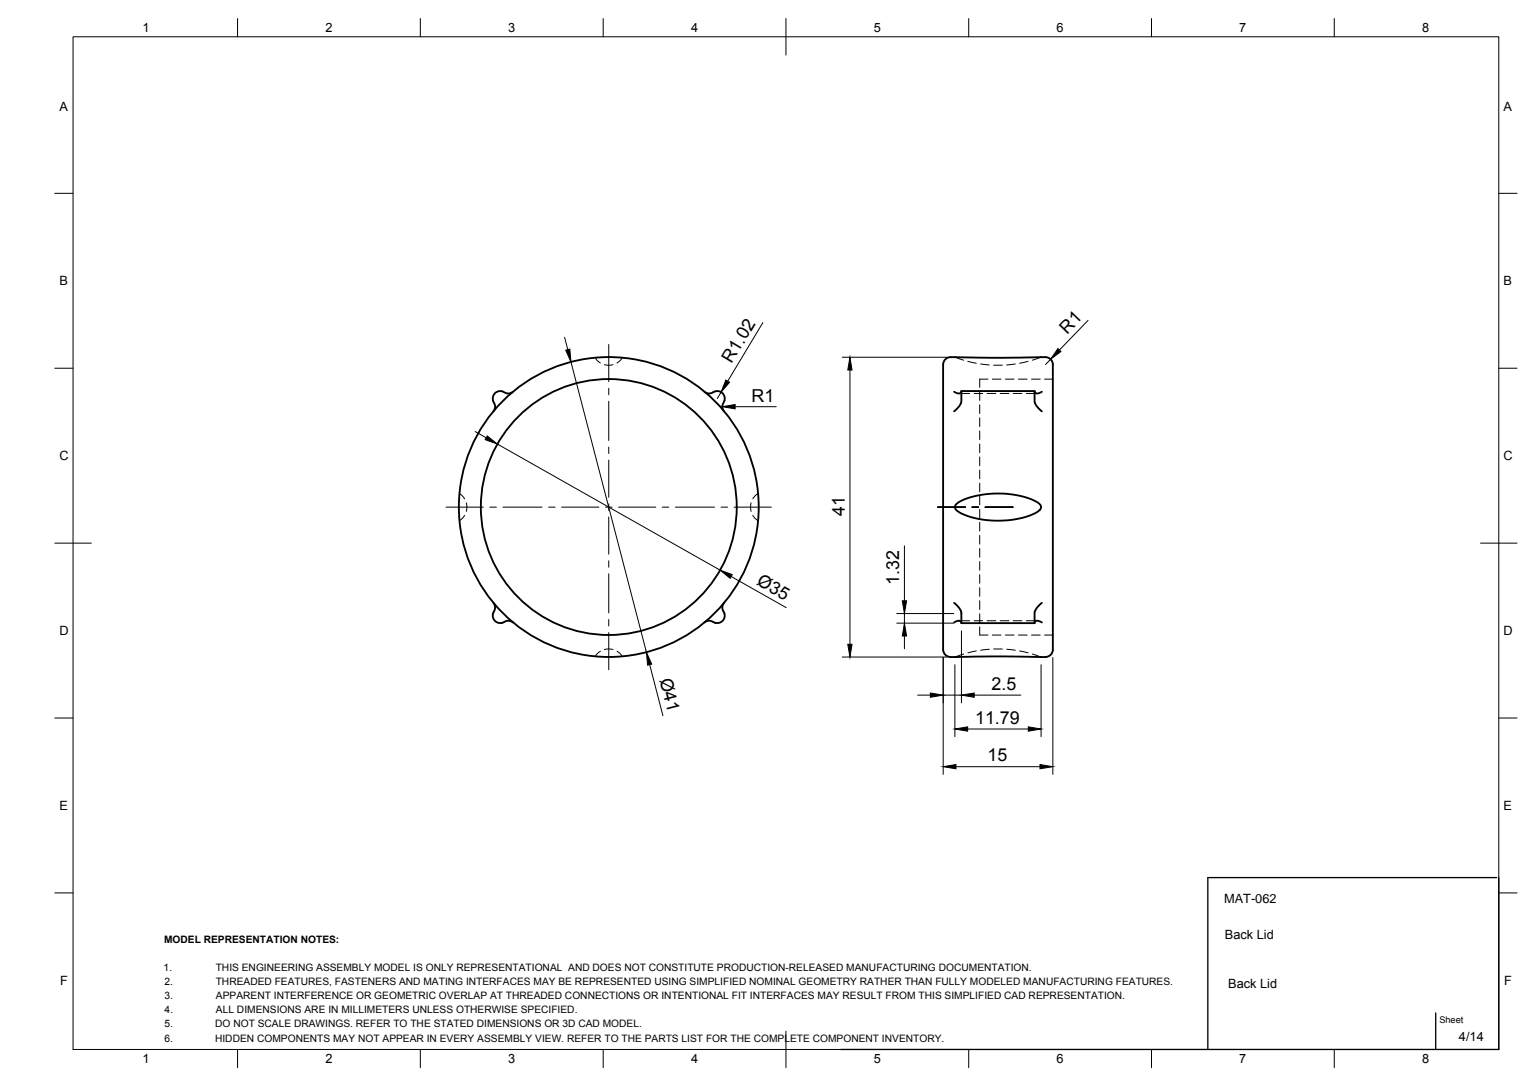
ISO-10303-21;
HEADER;
/* Generated by software containing ST-Developer
 * from STEP Tools, Inc. (www.steptools.com) 
 */

FILE_DESCRIPTION(
/* description */ (''),
/* implementation_level */ '2;1');

FILE_NAME(
/* name */ 'Back Lid.step',
/* time_stamp */ '2026-10-24T10:18:25-07:00',
/* author */ (''),
/* organization */ (''),
/* preprocessor_version */ 'ST-DEVELOPER v20.2',
/* originating_system */ 'Autodesk Translation Framework v15.15.0.0',
/* authorisation */ '');

FILE_SCHEMA (('AUTOMOTIVE_DESIGN { 1 0 10303 214 3 1 1 }'));
ENDSEC;

DATA;
#10=MECHANICAL_DESIGN_GEOMETRIC_PRESENTATION_REPRESENTATION('',(#248),#14125);
#199=TOROIDAL_SURFACE('',#6365,21.5,1.);
#200=TOROIDAL_SURFACE('',#6366,21.5,1.);
#201=TOROIDAL_SURFACE('',#6390,21.5,1.);
#202=TOROIDAL_SURFACE('',#6391,21.5,1.);
#203=TOROIDAL_SURFACE('',#6394,21.5,1.);
#204=TOROIDAL_SURFACE('',#6395,21.5,1.);
#205=TOROIDAL_SURFACE('',#6398,21.5,1.);
#206=TOROIDAL_SURFACE('',#6399,21.5,1.);
#207=TOROIDAL_SURFACE('',#6401,19.5,1.);
#208=TOROIDAL_SURFACE('',#6403,19.5,1.);
#219=(
BOUNDED_SURFACE()
B_SPLINE_SURFACE(2,2,((#10435,#10436,#10437,#10438,#10439),(#10440,#10441,
#10442,#10443,#10444),(#10445,#10446,#10447,#10448,#10449)),
 .UNSPECIFIED.,.F.,.F.,.F.)
B_SPLINE_SURFACE_WITH_KNOTS((3,3),(3,2,3),(-0.372145961557786,0.372122372471418),
(-2.5862005619648,-1.57539112175776,-0.564581681550713),.UNSPECIFIED.)
GEOMETRIC_REPRESENTATION_ITEM()
RATIONAL_B_SPLINE_SURFACE(((1.,0.874978596158143,1.,0.874978596158143,1.),
(0.931553475244656,0.815089352015808,0.931553475244656,0.815089352015808,
0.931553475244656),(1.,0.874978596158143,1.,0.874978596158143,1.)))
REPRESENTATION_ITEM('')
SURFACE()
);
#220=(
BOUNDED_SURFACE()
B_SPLINE_SURFACE(2,2,((#10450,#10451,#10452,#10453,#10454),(#10455,#10456,
#10457,#10458,#10459),(#10460,#10461,#10462,#10463,#10464)),
 .UNSPECIFIED.,.F.,.F.,.F.)
B_SPLINE_SURFACE_WITH_KNOTS((3,3),(3,2,3),(-0.372145961557785,0.372122372471416),
(-1.01540423516984,-0.00459479496282911,1.00621464524418),.UNSPECIFIED.)
GEOMETRIC_REPRESENTATION_ITEM()
RATIONAL_B_SPLINE_SURFACE(((1.,0.874978596158151,1.,0.874978596158151,1.),
(0.931553475244656,0.815089352015816,0.931553475244656,0.815089352015816,
0.931553475244656),(1.,0.874978596158151,1.,0.874978596158151,1.)))
REPRESENTATION_ITEM('')
SURFACE()
);
#221=(
BOUNDED_SURFACE()
B_SPLINE_SURFACE(2,2,((#10465,#10466,#10467,#10468,#10469),(#10470,#10471,
#10472,#10473,#10474),(#10475,#10476,#10477,#10478,#10479)),
 .UNSPECIFIED.,.F.,.F.,.F.)
B_SPLINE_SURFACE_WITH_KNOTS((3,3),(3,2,3),(-0.372145961557786,0.372122372471418),
(0.555392091624955,1.56620153183202,2.57701097203908),.UNSPECIFIED.)
GEOMETRIC_REPRESENTATION_ITEM()
RATIONAL_B_SPLINE_SURFACE(((1.,0.874978596158138,1.,0.874978596158138,1.),
(0.931553475244654,0.815089352015803,0.931553475244654,0.815089352015803,
0.931553475244654),(1.,0.874978596158138,1.,0.874978596158138,1.)))
REPRESENTATION_ITEM('')
SURFACE()
);
#222=(
BOUNDED_SURFACE()
B_SPLINE_SURFACE(2,2,((#10480,#10481,#10482,#10483,#10484),(#10485,#10486,
#10487,#10488,#10489),(#10490,#10491,#10492,#10493,#10494)),
 .UNSPECIFIED.,.F.,.F.,.F.)
B_SPLINE_SURFACE_WITH_KNOTS((3,3),(3,2,3),(-0.371934671474245,0.371934671474244),
(-1.01080944020701,0.,1.01080944020701),.UNSPECIFIED.)
GEOMETRIC_REPRESENTATION_ITEM()
RATIONAL_B_SPLINE_SURFACE(((1.,0.87497859615815,1.,0.87497859615815,1.),
(0.93162599415309,0.815152804508512,0.93162599415309,0.815152804508512,
0.93162599415309),(1.,0.87497859615815,1.,0.87497859615815,1.)))
REPRESENTATION_ITEM('')
SURFACE()
);
#228=SHAPE_REPRESENTATION_RELATIONSHIP('SRR','None',#14201,#238);
#238=ADVANCED_BREP_SHAPE_REPRESENTATION('',(#267),#14115);
#248=STYLED_ITEM('',(#14263),#267);
#267=MANIFOLD_SOLID_BREP('Back Lid',#6135);
#319=B_SPLINE_CURVE_WITH_KNOTS('',3,(#10199,#10200,#10201,#10202,#10203,
#10204,#10205,#10206),.UNSPECIFIED.,.F.,.F.,(4,2,2,4),(-1.01270550863141,
-0.972225883052009,-0.93592471729076,-0.9302261633243),.UNSPECIFIED.);
#320=B_SPLINE_CURVE_WITH_KNOTS('',3,(#10208,#10209,#10210,#10211,#10212,
#10213,#10214,#10215,#10216,#10217,#10218,#10219,#10220,#10221,#10222,#10223,
#10224,#10225,#10226,#10227,#10228,#10229),.UNSPECIFIED.,.F.,.F.,(4,2,2,
2,2,2,2,2,2,2,4),(0.770301299294677,0.776837516381544,0.810179859704117,
0.863854547164407,0.965601485426607,1.16658222290299,1.71041595764289,2.04547866914785,
2.21675572625692,2.31744906128486,2.32707423972487),.UNSPECIFIED.);
#321=B_SPLINE_CURVE_WITH_KNOTS('',3,(#10235,#10236,#10237,#10238,#10239,
#10240,#10241,#10242,#10243,#10244,#10245,#10246,#10247,#10248,#10249,#10250,
#10251,#10252,#10253,#10254,#10255,#10256,#10257,#10258,#10259),
 .UNSPECIFIED.,.F.,.F.,(4,2,2,2,2,3,2,2,2,2,2,4),(-0.9302261633243,-0.897559179923855,
-0.841033612998941,-0.72014052841894,-0.534875041413907,0.,0.287237711284631,
0.543909079429507,0.657892073847931,0.715678915934471,0.748705009105826,
0.770301299294677),.UNSPECIFIED.);
#322=B_SPLINE_CURVE_WITH_KNOTS('',3,(#10293,#10294,#10295,#10296,#10297,
#10298,#10299,#10300,#10301,#10302,#10303,#10304,#10305,#10306,#10307,#10308,
#10309,#10310,#10311,#10312,#10313,#10314,#10315,#10316,#10317,#10318,#10319,
#10320,#10321,#10322,#10323,#10324,#10325,#10326,#10327,#10328,#10329,#10330,
#10331,#10332,#10333,#10334,#10335,#10336),.UNSPECIFIED.,.T.,.F.,(4,2,2,
2,2,2,2,2,2,2,2,2,2,2,2,2,2,2,2,2,2,4),(-3.33977974833692,-3.05254203705232,
-2.79587066890727,-2.68188767448872,-2.62410083240212,-2.59107473923068,
-2.56294223195498,-2.52959988863245,-2.47592520117237,-2.37417826291126,
-2.17319752543706,-1.62936379070288,-1.29430107920164,-1.12302402209434,
-1.02233068706724,-0.972225883048282,-0.935924717287512,-0.897559179921191,
-0.841033612997187,-0.720140528418584,-0.534875041413949,0.),
 .UNSPECIFIED.);
#323=B_SPLINE_CURVE_WITH_KNOTS('',3,(#10338,#10339,#10340,#10341,#10342,
#10343,#10344,#10345,#10346,#10347,#10348,#10349,#10350,#10351,#10352,#10353,
#10354,#10355,#10356,#10357,#10358,#10359,#10360,#10361,#10362,#10363,#10364,
#10365,#10366,#10367,#10368,#10369,#10370,#10371,#10372,#10373,#10374,#10375,
#10376,#10377,#10378,#10379,#10380,#10381),.UNSPECIFIED.,.T.,.F.,(4,2,2,
2,2,2,2,2,2,2,2,2,2,2,2,2,2,2,2,2,2,4),(-3.3397797483622,-3.05254203707762,
-2.79587066893242,-2.68188767451365,-2.62410083242683,-2.5910747392553,
-2.5629422319795,-2.52959988865681,-2.47592520119621,-2.37417826293345,
-2.17319752545607,-1.62936379071395,-1.29430107920719,-1.1230240220981,
-1.02233068707054,-0.972225883051298,-0.93592471729009,-0.89755917992317,
-0.841033612998203,-0.720140528418294,-0.534875041413579,0.),
 .UNSPECIFIED.);
#324=B_SPLINE_CURVE_WITH_KNOTS('',3,(#10383,#10384,#10385,#10386,#10387,
#10388,#10389,#10390,#10391,#10392,#10393,#10394,#10395,#10396,#10397,#10398,
#10399,#10400,#10401,#10402,#10403,#10404,#10405,#10406,#10407,#10408,#10409,
#10410,#10411,#10412,#10413,#10414,#10415,#10416,#10417,#10418,#10419,#10420,
#10421,#10422,#10423,#10424,#10425,#10426),.UNSPECIFIED.,.T.,.F.,(4,2,2,
2,2,2,2,2,2,2,2,2,2,2,2,2,2,2,2,2,2,4),(-3.3397797483903,-3.05254203710569,
-2.79587066896086,-2.68188767454252,-2.62410083245608,-2.59107473928483,
-2.56294223200934,-2.52959988868709,-2.47592520122646,-2.37417826296174,
-2.17319752548078,-1.62936379072977,-1.29430107921846,-1.12302402210607,
-1.02233068707609,-0.972225883055856,-0.935924717293985,-0.897559179926439,
-0.841033613000712,-0.720140528419696,-0.534875041414283,0.),
 .UNSPECIFIED.);
#325=B_SPLINE_CURVE_WITH_KNOTS('',3,(#10500,#10501,#10502,#10503,#10504,
#10505),.UNSPECIFIED.,.F.,.F.,(4,2,4),(0.661047189651573,0.682893822496354,
0.69260663288377),.UNSPECIFIED.);
#326=B_SPLINE_CURVE_WITH_KNOTS('',3,(#10509,#10510,#10511,#10512,#10513,
#10514),.UNSPECIFIED.,.F.,.F.,(4,2,4),(0.954385955540414,0.955688960187291,
0.983990255335198),.UNSPECIFIED.);
#327=B_SPLINE_CURVE_WITH_KNOTS('',3,(#10518,#10519,#10520,#10521,#10522,
#10523),.UNSPECIFIED.,.F.,.F.,(4,2,4),(0.11431583352954,0.135832218753253,
0.145774815807224),.UNSPECIFIED.);
#328=B_SPLINE_CURVE_WITH_KNOTS('',3,(#10526,#10527,#10528,#10529,#10530,
#10531),.UNSPECIFIED.,.F.,.F.,(4,2,4),(0.406957049146252,0.408029153839697,
0.43652027355868),.UNSPECIFIED.);
#329=B_SPLINE_CURVE_WITH_KNOTS('',3,(#10537,#10538,#10539,#10540,#10541,
#10542,#10543,#10544,#10545,#10546),.UNSPECIFIED.,.F.,.F.,(4,2,2,2,4),(-0.178698063821344,
-0.13526955955559,-0.076624980274606,0.,0.000624348927189005),
 .UNSPECIFIED.);
#330=B_SPLINE_CURVE_WITH_KNOTS('',3,(#10547,#10548,#10549,#10550,#10551,
#10552,#10553,#10554,#10555,#10556),.UNSPECIFIED.,.F.,.F.,(4,2,2,2,4),(0.221433756193381,
0.257003031040665,0.305034737267452,0.367792942517405,0.3683043034075),
 .UNSPECIFIED.);
#331=B_SPLINE_CURVE_WITH_KNOTS('',3,(#10558,#10559,#10560,#10561,#10562,
#10563,#10564,#10565,#10566,#10567),.UNSPECIFIED.,.F.,.F.,(4,2,2,2,4),(-0.178698063657826,
-0.135269559443281,-0.0766249802302674,0.,0.000624348926984052),
 .UNSPECIFIED.);
#332=B_SPLINE_CURVE_WITH_KNOTS('',3,(#10569,#10570,#10571,#10572,#10573,
#10574,#10575,#10576,#10577,#10578),.UNSPECIFIED.,.F.,.F.,(4,2,2,2,4),(0.22143375619356,
0.257003031040236,0.305034737266783,0.367792942534155,0.36830430342492),
 .UNSPECIFIED.);
#333=B_SPLINE_CURVE_WITH_KNOTS('',3,(#10585,#10586,#10587,#10588,#10589,
#10590),.UNSPECIFIED.,.F.,.F.,(4,2,4),(0.661047189631137,0.682893822475484,
0.692606632862655),.UNSPECIFIED.);
#334=B_SPLINE_CURVE_WITH_KNOTS('',3,(#10594,#10595,#10596,#10597,#10598,
#10599),.UNSPECIFIED.,.F.,.F.,(4,2,4),(0.954385955875588,0.955688960523108,
0.983990255684603),.UNSPECIFIED.);
#335=B_SPLINE_CURVE_WITH_KNOTS('',3,(#10603,#10604,#10605,#10606,#10607,
#10608),.UNSPECIFIED.,.F.,.F.,(4,2,4),(0.11431583355748,0.135832218786672,
0.145774815843186),.UNSPECIFIED.);
#336=B_SPLINE_CURVE_WITH_KNOTS('',3,(#10611,#10612,#10613,#10614,#10615,
#10616),.UNSPECIFIED.,.F.,.F.,(4,2,4),(0.406957049130622,0.408029153824045,
0.436520273542523),.UNSPECIFIED.);
#337=B_SPLINE_CURVE_WITH_KNOTS('',3,(#10626,#10627,#10628,#10629,#10630,
#10631),.UNSPECIFIED.,.F.,.F.,(4,2,4),(0.661047189621191,0.682893822464398,
0.692606632851314),.UNSPECIFIED.);
#338=B_SPLINE_CURVE_WITH_KNOTS('',3,(#10635,#10636,#10637,#10638,#10639,
#10640),.UNSPECIFIED.,.F.,.F.,(4,2,4),(0.954385955650832,0.95568896029806,
0.983990255452134),.UNSPECIFIED.);
#339=B_SPLINE_CURVE_WITH_KNOTS('',3,(#10644,#10645,#10646,#10647,#10648,
#10649),.UNSPECIFIED.,.F.,.F.,(4,2,4),(0.114315833531678,0.135832218756235,
0.145774815810657),.UNSPECIFIED.);
#340=B_SPLINE_CURVE_WITH_KNOTS('',3,(#10652,#10653,#10654,#10655,#10656,
#10657),.UNSPECIFIED.,.F.,.F.,(4,2,4),(0.406957049123385,0.408029153816832,
0.43652027353595),.UNSPECIFIED.);
#341=B_SPLINE_CURVE_WITH_KNOTS('',3,(#10667,#10668,#10669,#10670,#10671,
#10672),.UNSPECIFIED.,.F.,.F.,(4,2,4),(0.661047189700789,0.682893822549002,
0.692606632937976),.UNSPECIFIED.);
#342=B_SPLINE_CURVE_WITH_KNOTS('',3,(#10676,#10677,#10678,#10679,#10680,
#10681),.UNSPECIFIED.,.F.,.F.,(4,2,4),(0.954385955972242,0.955688960619816,
0.983990255786846),.UNSPECIFIED.);
#343=B_SPLINE_CURVE_WITH_KNOTS('',3,(#10685,#10686,#10687,#10688,#10689,
#10690),.UNSPECIFIED.,.F.,.F.,(4,2,4),(0.114315833560946,0.135832218791008,
0.145774815847966),.UNSPECIFIED.);
#344=B_SPLINE_CURVE_WITH_KNOTS('',3,(#10693,#10694,#10695,#10696,#10697,
#10698),.UNSPECIFIED.,.F.,.F.,(4,2,4),(0.406957049170082,0.408029153863569,
0.436520273584039),.UNSPECIFIED.);
#345=B_SPLINE_CURVE_WITH_KNOTS('',3,(#10704,#10705,#10706,#10707,#10708,
#10709,#10710,#10711,#10712,#10713),.UNSPECIFIED.,.F.,.F.,(4,2,2,2,4),(-0.17869806353704,
-0.135269559359834,-0.0766249801970823,0.,0.000624348926732177),
 .UNSPECIFIED.);
#346=B_SPLINE_CURVE_WITH_KNOTS('',3,(#10714,#10715,#10716,#10717,#10718,
#10719,#10720,#10721,#10722,#10723),.UNSPECIFIED.,.F.,.F.,(4,2,2,2,4),(0.221433756192697,
0.257003031038445,0.305034737264325,0.3677929425703,0.368304303461073),
 .UNSPECIFIED.);
#347=B_SPLINE_CURVE_WITH_KNOTS('',3,(#10725,#10726,#10727,#10728,#10729,
#10730,#10731,#10732,#10733,#10734),.UNSPECIFIED.,.F.,.F.,(4,2,2,2,4),(-0.178698063770044,
-0.135269559520182,-0.0766249802604931,0.,0.000624348926843672),
 .UNSPECIFIED.);
#348=B_SPLINE_CURVE_WITH_KNOTS('',3,(#10736,#10737,#10738,#10739,#10740,
#10741,#10742,#10743,#10744,#10745),.UNSPECIFIED.,.F.,.F.,(4,2,2,2,4),(0.221433756193478,
0.257003031040149,0.305034737266569,0.367792942538401,0.368304303428461),
 .UNSPECIFIED.);
#349=B_SPLINE_CURVE_WITH_KNOTS('',3,(#10748,#10749,#10750,#10751,#10752,
#10753,#10754,#10755,#10756,#10757),.UNSPECIFIED.,.F.,.F.,(4,2,2,2,4),(-0.178698063553284,
-0.135269559371072,-0.0766249802015666,0.,0.000624348926677296),
 .UNSPECIFIED.);
#350=B_SPLINE_CURVE_WITH_KNOTS('',3,(#10758,#10759,#10760,#10761,#10762,
#10763,#10764,#10765,#10766,#10767),.UNSPECIFIED.,.F.,.F.,(4,2,2,2,4),(0.221433756192838,
0.25700303103897,0.305034737265084,0.367792942555533,0.368304303445851),
 .UNSPECIFIED.);
#351=B_SPLINE_CURVE_WITH_KNOTS('',3,(#10769,#10770,#10771,#10772,#10773,
#10774,#10775,#10776,#10777,#10778),.UNSPECIFIED.,.F.,.F.,(4,2,2,2,4),(-0.178698063553173,
-0.135269559370956,-0.0766249802014978,0.,0.000624348926817562),
 .UNSPECIFIED.);
#352=B_SPLINE_CURVE_WITH_KNOTS('',3,(#10780,#10781,#10782,#10783,#10784,
#10785,#10786,#10787,#10788,#10789),.UNSPECIFIED.,.F.,.F.,(4,2,2,2,4),(0.221433756193333,
0.25700303103906,0.305034737264906,0.367792942572609,0.368304303463133),
 .UNSPECIFIED.);
#353=B_SPLINE_CURVE_WITH_KNOTS('',3,(#10792,#10793,#10794,#10795,#10796,
#10797,#10798,#10799,#10800,#10801),.UNSPECIFIED.,.F.,.F.,(4,2,2,2,4),(-0.178698063530463,
-0.135269559355353,-0.0766249801953056,0.,0.000624348926771406),
 .UNSPECIFIED.);
#354=B_SPLINE_CURVE_WITH_KNOTS('',3,(#10802,#10803,#10804,#10805,#10806,
#10807,#10808,#10809,#10810,#10811),.UNSPECIFIED.,.F.,.F.,(4,2,2,2,4),(0.221433756193692,
0.2570030310401,0.30503473726647,0.367792942548679,0.368304303439319),
 .UNSPECIFIED.);
#355=B_SPLINE_CURVE_WITH_KNOTS('',3,(#10813,#10814,#10815,#10816,#10817,
#10818,#10819,#10820,#10821,#10822),.UNSPECIFIED.,.F.,.F.,(4,2,2,2,4),(-0.178698063395802,
-0.135269559262804,-0.0766249801587596,0.,0.00062434892634055),
 .UNSPECIFIED.);
#356=B_SPLINE_CURVE_WITH_KNOTS('',3,(#10824,#10825,#10826,#10827,#10828,
#10829,#10830,#10831,#10832,#10833),.UNSPECIFIED.,.F.,.F.,(4,2,2,2,4),(0.221433756192834,
0.257003031038388,0.305034737264263,0.367792942576978,0.368304303467952),
 .UNSPECIFIED.);
#499=CYLINDRICAL_SURFACE('',#6339,20.5);
#500=CYLINDRICAL_SURFACE('',#6357,1.02425693042952);
#501=CYLINDRICAL_SURFACE('',#6364,1.);
#502=CYLINDRICAL_SURFACE('',#6367,1.);
#503=CYLINDRICAL_SURFACE('',#6368,1.02425693042952);
#504=CYLINDRICAL_SURFACE('',#6375,1.02425693042952);
#505=CYLINDRICAL_SURFACE('',#6382,1.02425693042952);
#506=CYLINDRICAL_SURFACE('',#6389,1.);
#507=CYLINDRICAL_SURFACE('',#6392,1.);
#508=CYLINDRICAL_SURFACE('',#6393,1.);
#509=CYLINDRICAL_SURFACE('',#6396,1.);
#510=CYLINDRICAL_SURFACE('',#6397,1.);
#511=CYLINDRICAL_SURFACE('',#6400,1.);
#512=CYLINDRICAL_SURFACE('',#6405,17.5);
#646=FACE_BOUND('',#1156,.T.);
#647=FACE_BOUND('',#1157,.T.);
#648=FACE_BOUND('',#1158,.T.);
#649=FACE_BOUND('',#1159,.T.);
#650=FACE_BOUND('',#1160,.T.);
#651=FACE_BOUND('',#1161,.T.);
#652=FACE_BOUND('',#1162,.T.);
#653=FACE_BOUND('',#1165,.T.);
#783=FACE_OUTER_BOUND('',#1155,.T.);
#784=FACE_OUTER_BOUND('',#1163,.T.);
#785=FACE_OUTER_BOUND('',#1164,.T.);
#786=FACE_OUTER_BOUND('',#1166,.T.);
#787=FACE_OUTER_BOUND('',#1167,.T.);
#788=FACE_OUTER_BOUND('',#1168,.T.);
#789=FACE_OUTER_BOUND('',#1169,.T.);
#790=FACE_OUTER_BOUND('',#1170,.T.);
#791=FACE_OUTER_BOUND('',#1171,.T.);
#792=FACE_OUTER_BOUND('',#1172,.T.);
#793=FACE_OUTER_BOUND('',#1173,.T.);
#794=FACE_OUTER_BOUND('',#1174,.T.);
#795=FACE_OUTER_BOUND('',#1175,.T.);
#796=FACE_OUTER_BOUND('',#1176,.T.);
#797=FACE_OUTER_BOUND('',#1177,.T.);
#798=FACE_OUTER_BOUND('',#1178,.T.);
#799=FACE_OUTER_BOUND('',#1179,.T.);
#800=FACE_OUTER_BOUND('',#1180,.T.);
#801=FACE_OUTER_BOUND('',#1181,.T.);
#802=FACE_OUTER_BOUND('',#1182,.T.);
#803=FACE_OUTER_BOUND('',#1183,.T.);
#804=FACE_OUTER_BOUND('',#1184,.T.);
#805=FACE_OUTER_BOUND('',#1185,.T.);
#806=FACE_OUTER_BOUND('',#1186,.T.);
#807=FACE_OUTER_BOUND('',#1187,.T.);
#808=FACE_OUTER_BOUND('',#1188,.T.);
#809=FACE_OUTER_BOUND('',#1189,.T.);
#810=FACE_OUTER_BOUND('',#1190,.T.);
#811=FACE_OUTER_BOUND('',#1191,.T.);
#812=FACE_OUTER_BOUND('',#1192,.T.);
#813=FACE_OUTER_BOUND('',#1193,.T.);
#814=FACE_OUTER_BOUND('',#1194,.T.);
#815=FACE_OUTER_BOUND('',#1195,.T.);
#816=FACE_OUTER_BOUND('',#1196,.T.);
#817=FACE_OUTER_BOUND('',#1197,.T.);
#818=FACE_OUTER_BOUND('',#1198,.T.);
#819=FACE_OUTER_BOUND('',#1199,.T.);
#820=FACE_OUTER_BOUND('',#1200,.T.);
#821=FACE_OUTER_BOUND('',#1201,.T.);
#1155=EDGE_LOOP('',(#4221,#4222,#4223,#4224,#4225,#4226,#4227,#4228,#4229,
#4230,#4231));
#1156=EDGE_LOOP('',(#4232,#4233,#4234,#4235));
#1157=EDGE_LOOP('',(#4236,#4237,#4238,#4239));
#1158=EDGE_LOOP('',(#4240,#4241,#4242,#4243));
#1159=EDGE_LOOP('',(#4244,#4245,#4246,#4247));
#1160=EDGE_LOOP('',(#4248));
#1161=EDGE_LOOP('',(#4249));
#1162=EDGE_LOOP('',(#4250));
#1163=EDGE_LOOP('',(#4251));
#1164=EDGE_LOOP('',(#4252));
#1165=EDGE_LOOP('',(#4253));
#1166=EDGE_LOOP('',(#4254));
#1167=EDGE_LOOP('',(#4255));
#1168=EDGE_LOOP('',(#4256));
#1169=EDGE_LOOP('',(#4257,#4258,#4259));
#1170=EDGE_LOOP('',(#4260,#4261,#4262,#4263,#4264,#4265,#4266,#4267));
#1171=EDGE_LOOP('',(#4268,#4269));
#1172=EDGE_LOOP('',(#4270,#4271));
#1173=EDGE_LOOP('',(#4272,#4273,#4274,#4275));
#1174=EDGE_LOOP('',(#4276,#4277,#4278,#4279,#4280,#4281));
#1175=EDGE_LOOP('',(#4282,#4283,#4284,#4285,#4286,#4287));
#1176=EDGE_LOOP('',(#4288,#4289,#4290,#4291));
#1177=EDGE_LOOP('',(#4292,#4293,#4294,#4295,#4296,#4297,#4298,#4299));
#1178=EDGE_LOOP('',(#4300,#4301));
#1179=EDGE_LOOP('',(#4302,#4303));
#1180=EDGE_LOOP('',(#4304,#4305,#4306,#4307,#4308,#4309,#4310,#4311));
#1181=EDGE_LOOP('',(#4312,#4313));
#1182=EDGE_LOOP('',(#4314,#4315));
#1183=EDGE_LOOP('',(#4316,#4317,#4318,#4319,#4320,#4321,#4322,#4323));
#1184=EDGE_LOOP('',(#4324,#4325));
#1185=EDGE_LOOP('',(#4326,#4327));
#1186=EDGE_LOOP('',(#4328,#4329,#4330,#4331));
#1187=EDGE_LOOP('',(#4332,#4333,#4334,#4335,#4336,#4337));
#1188=EDGE_LOOP('',(#4338,#4339,#4340,#4341,#4342,#4343));
#1189=EDGE_LOOP('',(#4344,#4345,#4346,#4347));
#1190=EDGE_LOOP('',(#4348,#4349,#4350,#4351));
#1191=EDGE_LOOP('',(#4352,#4353,#4354,#4355,#4356,#4357));
#1192=EDGE_LOOP('',(#4358,#4359,#4360,#4361,#4362,#4363));
#1193=EDGE_LOOP('',(#4364,#4365,#4366,#4367));
#1194=EDGE_LOOP('',(#4368,#4369,#4370,#4371));
#1195=EDGE_LOOP('',(#4372,#4373,#4374,#4375,#4376,#4377));
#1196=EDGE_LOOP('',(#4378,#4379,#4380,#4381,#4382,#4383));
#1197=EDGE_LOOP('',(#4384,#4385,#4386,#4387));
#1198=EDGE_LOOP('',(#4388,#4389,#4390,#4391,#4392));
#1199=EDGE_LOOP('',(#4393,#4394,#4395,#4396,#4397));
#1200=EDGE_LOOP('',(#4398,#4399,#4400,#4401));
#1201=EDGE_LOOP('',(#4402));
#1580=CIRCLE('',#6340,20.5);
#1581=CIRCLE('',#6341,20.5);
#1582=CIRCLE('',#6342,20.5);
#1583=CIRCLE('',#6343,20.5);
#1584=CIRCLE('',#6344,20.5);
#1585=CIRCLE('',#6345,20.5);
#1586=CIRCLE('',#6346,20.5);
#1587=CIRCLE('',#6347,20.5);
#1588=CIRCLE('',#6348,20.5);
#1589=CIRCLE('',#6349,20.5);
#1590=CIRCLE('',#6350,20.5);
#1591=CIRCLE('',#6351,20.5);
#1592=CIRCLE('',#6353,19.5);
#1593=CIRCLE('',#6355,19.5);
#1594=CIRCLE('',#6356,17.5);
#1595=CIRCLE('',#6358,1.02425693042952);
#1596=CIRCLE('',#6359,1.02425693042952);
#1597=CIRCLE('',#6361,21.5);
#1598=CIRCLE('',#6363,21.5);
#1599=CIRCLE('',#6369,1.02425693042952);
#1600=CIRCLE('',#6370,1.02425693042952);
#1601=CIRCLE('',#6372,21.5);
#1602=CIRCLE('',#6374,21.5);
#1603=CIRCLE('',#6376,1.02425693042952);
#1604=CIRCLE('',#6377,1.02425693042952);
#1605=CIRCLE('',#6379,21.5);
#1606=CIRCLE('',#6381,21.5);
#1607=CIRCLE('',#6383,1.02425693042952);
#1608=CIRCLE('',#6384,1.02425693042952);
#1609=CIRCLE('',#6386,21.5);
#1610=CIRCLE('',#6388,21.5);
#1611=CIRCLE('',#6402,1.);
#1612=CIRCLE('',#6404,1.);
#1613=CIRCLE('',#6406,17.5);
#1869=LINE('',#10197,#2257);
#1870=LINE('',#10231,#2258);
#1871=LINE('',#10262,#2259);
#1872=LINE('',#10266,#2260);
#1873=LINE('',#10270,#2261);
#1874=LINE('',#10274,#2262);
#1875=LINE('',#10278,#2263);
#1876=LINE('',#10282,#2264);
#1877=LINE('',#10286,#2265);
#1878=LINE('',#10290,#2266);
#1879=LINE('',#10507,#2267);
#1880=LINE('',#10525,#2268);
#1881=LINE('',#10592,#2269);
#1882=LINE('',#10610,#2270);
#1883=LINE('',#10633,#2271);
#1884=LINE('',#10651,#2272);
#1885=LINE('',#10674,#2273);
#1886=LINE('',#10692,#2274);
#1887=LINE('',#10841,#2275);
#2257=VECTOR('',#7141,20.5);
#2258=VECTOR('',#7142,20.5);
#2259=VECTOR('',#7147,12.);
#2260=VECTOR('',#7150,12.);
#2261=VECTOR('',#7153,12.);
#2262=VECTOR('',#7156,12.);
#2263=VECTOR('',#7159,12.);
#2264=VECTOR('',#7162,12.);
#2265=VECTOR('',#7165,12.);
#2266=VECTOR('',#7168,12.);
#2267=VECTOR('',#7185,10.0757988598381);
#2268=VECTOR('',#7188,10.0757988598381);
#2269=VECTOR('',#7209,10.0757988598381);
#2270=VECTOR('',#7212,10.0757988598381);
#2271=VECTOR('',#7225,10.0757988598381);
#2272=VECTOR('',#7228,10.0757988598381);
#2273=VECTOR('',#7241,10.0757988598381);
#2274=VECTOR('',#7244,10.0757988598381);
#2275=VECTOR('',#7287,17.5);
#2659=VERTEX_POINT('',#10192);
#2660=VERTEX_POINT('',#10193);
#2661=VERTEX_POINT('',#10196);
#2662=VERTEX_POINT('',#10198);
#2663=VERTEX_POINT('',#10207);
#2664=VERTEX_POINT('',#10230);
#2665=VERTEX_POINT('',#10232);
#2666=VERTEX_POINT('',#10260);
#2667=VERTEX_POINT('',#10261);
#2668=VERTEX_POINT('',#10263);
#2669=VERTEX_POINT('',#10265);
#2670=VERTEX_POINT('',#10268);
#2671=VERTEX_POINT('',#10269);
#2672=VERTEX_POINT('',#10271);
#2673=VERTEX_POINT('',#10273);
#2674=VERTEX_POINT('',#10276);
#2675=VERTEX_POINT('',#10277);
#2676=VERTEX_POINT('',#10279);
#2677=VERTEX_POINT('',#10281);
#2678=VERTEX_POINT('',#10284);
#2679=VERTEX_POINT('',#10285);
#2680=VERTEX_POINT('',#10287);
#2681=VERTEX_POINT('',#10289);
#2682=VERTEX_POINT('',#10292);
#2683=VERTEX_POINT('',#10337);
#2684=VERTEX_POINT('',#10382);
#2685=VERTEX_POINT('',#10428);
#2686=VERTEX_POINT('',#10431);
#2687=VERTEX_POINT('',#10433);
#2688=VERTEX_POINT('',#10496);
#2689=VERTEX_POINT('',#10497);
#2690=VERTEX_POINT('',#10499);
#2691=VERTEX_POINT('',#10506);
#2692=VERTEX_POINT('',#10508);
#2693=VERTEX_POINT('',#10515);
#2694=VERTEX_POINT('',#10517);
#2695=VERTEX_POINT('',#10524);
#2696=VERTEX_POINT('',#10581);
#2697=VERTEX_POINT('',#10582);
#2698=VERTEX_POINT('',#10584);
#2699=VERTEX_POINT('',#10591);
#2700=VERTEX_POINT('',#10593);
#2701=VERTEX_POINT('',#10600);
#2702=VERTEX_POINT('',#10602);
#2703=VERTEX_POINT('',#10609);
#2704=VERTEX_POINT('',#10622);
#2705=VERTEX_POINT('',#10623);
#2706=VERTEX_POINT('',#10625);
#2707=VERTEX_POINT('',#10632);
#2708=VERTEX_POINT('',#10634);
#2709=VERTEX_POINT('',#10641);
#2710=VERTEX_POINT('',#10643);
#2711=VERTEX_POINT('',#10650);
#2712=VERTEX_POINT('',#10663);
#2713=VERTEX_POINT('',#10664);
#2714=VERTEX_POINT('',#10666);
#2715=VERTEX_POINT('',#10673);
#2716=VERTEX_POINT('',#10675);
#2717=VERTEX_POINT('',#10682);
#2718=VERTEX_POINT('',#10684);
#2719=VERTEX_POINT('',#10691);
#2720=VERTEX_POINT('',#10840);
#3258=EDGE_CURVE('',#2659,#2660,#1580,.T.);
#3259=EDGE_CURVE('',#2660,#2659,#1581,.T.);
#3260=EDGE_CURVE('',#2659,#2661,#1869,.T.);
#3261=EDGE_CURVE('',#2662,#2661,#319,.T.);
#3262=EDGE_CURVE('',#2663,#2662,#320,.T.);
#3263=EDGE_CURVE('',#2663,#2664,#1870,.T.);
#3264=EDGE_CURVE('',#2664,#2665,#1582,.F.);
#3265=EDGE_CURVE('',#2665,#2664,#1583,.F.);
#3266=EDGE_CURVE('',#2661,#2663,#321,.T.);
#3267=EDGE_CURVE('',#2666,#2667,#1871,.F.);
#3268=EDGE_CURVE('',#2667,#2668,#1584,.T.);
#3269=EDGE_CURVE('',#2668,#2669,#1872,.T.);
#3270=EDGE_CURVE('',#2669,#2666,#1585,.F.);
#3271=EDGE_CURVE('',#2670,#2671,#1873,.F.);
#3272=EDGE_CURVE('',#2671,#2672,#1586,.T.);
#3273=EDGE_CURVE('',#2672,#2673,#1874,.T.);
#3274=EDGE_CURVE('',#2673,#2670,#1587,.F.);
#3275=EDGE_CURVE('',#2674,#2675,#1875,.F.);
#3276=EDGE_CURVE('',#2675,#2676,#1588,.T.);
#3277=EDGE_CURVE('',#2676,#2677,#1876,.T.);
#3278=EDGE_CURVE('',#2677,#2674,#1589,.F.);
#3279=EDGE_CURVE('',#2678,#2679,#1877,.F.);
#3280=EDGE_CURVE('',#2679,#2680,#1590,.T.);
#3281=EDGE_CURVE('',#2680,#2681,#1878,.T.);
#3282=EDGE_CURVE('',#2681,#2678,#1591,.F.);
#3283=EDGE_CURVE('',#2682,#2682,#322,.T.);
#3284=EDGE_CURVE('',#2683,#2683,#323,.T.);
#3285=EDGE_CURVE('',#2684,#2684,#324,.T.);
#3286=EDGE_CURVE('',#2685,#2685,#1592,.T.);
#3287=EDGE_CURVE('',#2686,#2686,#1593,.F.);
#3288=EDGE_CURVE('',#2687,#2687,#1594,.F.);
#3289=EDGE_CURVE('',#2688,#2689,#1595,.T.);
#3290=EDGE_CURVE('',#2688,#2690,#325,.T.);
#3291=EDGE_CURVE('',#2690,#2691,#1879,.T.);
#3292=EDGE_CURVE('',#2691,#2692,#326,.T.);
#3293=EDGE_CURVE('',#2692,#2693,#1596,.T.);
#3294=EDGE_CURVE('',#2693,#2694,#327,.T.);
#3295=EDGE_CURVE('',#2694,#2695,#1880,.F.);
#3296=EDGE_CURVE('',#2695,#2689,#328,.T.);
#3297=EDGE_CURVE('',#2689,#2688,#1597,.F.);
#3298=EDGE_CURVE('',#2692,#2693,#1598,.T.);
#3299=EDGE_CURVE('',#2681,#2694,#329,.F.);
#3300=EDGE_CURVE('',#2695,#2680,#330,.T.);
#3301=EDGE_CURVE('',#2690,#2679,#331,.T.);
#3302=EDGE_CURVE('',#2678,#2691,#332,.F.);
#3303=EDGE_CURVE('',#2696,#2697,#1599,.T.);
#3304=EDGE_CURVE('',#2696,#2698,#333,.T.);
#3305=EDGE_CURVE('',#2698,#2699,#1881,.T.);
#3306=EDGE_CURVE('',#2699,#2700,#334,.T.);
#3307=EDGE_CURVE('',#2700,#2701,#1600,.T.);
#3308=EDGE_CURVE('',#2701,#2702,#335,.T.);
#3309=EDGE_CURVE('',#2702,#2703,#1882,.F.);
#3310=EDGE_CURVE('',#2703,#2697,#336,.T.);
#3311=EDGE_CURVE('',#2697,#2696,#1601,.F.);
#3312=EDGE_CURVE('',#2700,#2701,#1602,.T.);
#3313=EDGE_CURVE('',#2704,#2705,#1603,.T.);
#3314=EDGE_CURVE('',#2704,#2706,#337,.T.);
#3315=EDGE_CURVE('',#2706,#2707,#1883,.T.);
#3316=EDGE_CURVE('',#2707,#2708,#338,.T.);
#3317=EDGE_CURVE('',#2708,#2709,#1604,.T.);
#3318=EDGE_CURVE('',#2709,#2710,#339,.T.);
#3319=EDGE_CURVE('',#2710,#2711,#1884,.F.);
#3320=EDGE_CURVE('',#2711,#2705,#340,.T.);
#3321=EDGE_CURVE('',#2705,#2704,#1605,.F.);
#3322=EDGE_CURVE('',#2708,#2709,#1606,.T.);
#3323=EDGE_CURVE('',#2712,#2713,#1607,.T.);
#3324=EDGE_CURVE('',#2712,#2714,#341,.T.);
#3325=EDGE_CURVE('',#2714,#2715,#1885,.T.);
#3326=EDGE_CURVE('',#2715,#2716,#342,.T.);
#3327=EDGE_CURVE('',#2716,#2717,#1608,.T.);
#3328=EDGE_CURVE('',#2717,#2718,#343,.T.);
#3329=EDGE_CURVE('',#2718,#2719,#1886,.F.);
#3330=EDGE_CURVE('',#2719,#2713,#344,.T.);
#3331=EDGE_CURVE('',#2713,#2712,#1609,.F.);
#3332=EDGE_CURVE('',#2716,#2717,#1610,.T.);
#3333=EDGE_CURVE('',#2677,#2718,#345,.F.);
#3334=EDGE_CURVE('',#2719,#2676,#346,.T.);
#3335=EDGE_CURVE('',#2714,#2675,#347,.T.);
#3336=EDGE_CURVE('',#2674,#2715,#348,.F.);
#3337=EDGE_CURVE('',#2673,#2710,#349,.F.);
#3338=EDGE_CURVE('',#2711,#2672,#350,.T.);
#3339=EDGE_CURVE('',#2706,#2671,#351,.T.);
#3340=EDGE_CURVE('',#2670,#2707,#352,.F.);
#3341=EDGE_CURVE('',#2669,#2702,#353,.F.);
#3342=EDGE_CURVE('',#2703,#2668,#354,.T.);
#3343=EDGE_CURVE('',#2698,#2667,#355,.T.);
#3344=EDGE_CURVE('',#2666,#2699,#356,.F.);
#3345=EDGE_CURVE('',#2660,#2686,#1611,.T.);
#3346=EDGE_CURVE('',#2685,#2665,#1612,.T.);
#3347=EDGE_CURVE('',#2687,#2720,#1887,.T.);
#3348=EDGE_CURVE('',#2720,#2720,#1613,.T.);
#4221=ORIENTED_EDGE('',*,*,#3258,.T.);
#4222=ORIENTED_EDGE('',*,*,#3259,.T.);
#4223=ORIENTED_EDGE('',*,*,#3260,.T.);
#4224=ORIENTED_EDGE('',*,*,#3261,.F.);
#4225=ORIENTED_EDGE('',*,*,#3262,.F.);
#4226=ORIENTED_EDGE('',*,*,#3263,.T.);
#4227=ORIENTED_EDGE('',*,*,#3264,.T.);
#4228=ORIENTED_EDGE('',*,*,#3265,.T.);
#4229=ORIENTED_EDGE('',*,*,#3263,.F.);
#4230=ORIENTED_EDGE('',*,*,#3266,.F.);
#4231=ORIENTED_EDGE('',*,*,#3260,.F.);
#4232=ORIENTED_EDGE('',*,*,#3267,.T.);
#4233=ORIENTED_EDGE('',*,*,#3268,.T.);
#4234=ORIENTED_EDGE('',*,*,#3269,.T.);
#4235=ORIENTED_EDGE('',*,*,#3270,.T.);
#4236=ORIENTED_EDGE('',*,*,#3271,.T.);
#4237=ORIENTED_EDGE('',*,*,#3272,.T.);
#4238=ORIENTED_EDGE('',*,*,#3273,.T.);
#4239=ORIENTED_EDGE('',*,*,#3274,.T.);
#4240=ORIENTED_EDGE('',*,*,#3275,.T.);
#4241=ORIENTED_EDGE('',*,*,#3276,.T.);
#4242=ORIENTED_EDGE('',*,*,#3277,.T.);
#4243=ORIENTED_EDGE('',*,*,#3278,.T.);
#4244=ORIENTED_EDGE('',*,*,#3279,.T.);
#4245=ORIENTED_EDGE('',*,*,#3280,.T.);
#4246=ORIENTED_EDGE('',*,*,#3281,.T.);
#4247=ORIENTED_EDGE('',*,*,#3282,.T.);
#4248=ORIENTED_EDGE('',*,*,#3283,.F.);
#4249=ORIENTED_EDGE('',*,*,#3284,.F.);
#4250=ORIENTED_EDGE('',*,*,#3285,.F.);
#4251=ORIENTED_EDGE('',*,*,#3286,.T.);
#4252=ORIENTED_EDGE('',*,*,#3287,.T.);
#4253=ORIENTED_EDGE('',*,*,#3288,.F.);
#4254=ORIENTED_EDGE('',*,*,#3283,.T.);
#4255=ORIENTED_EDGE('',*,*,#3284,.T.);
#4256=ORIENTED_EDGE('',*,*,#3285,.T.);
#4257=ORIENTED_EDGE('',*,*,#3261,.T.);
#4258=ORIENTED_EDGE('',*,*,#3266,.T.);
#4259=ORIENTED_EDGE('',*,*,#3262,.T.);
#4260=ORIENTED_EDGE('',*,*,#3289,.F.);
#4261=ORIENTED_EDGE('',*,*,#3290,.T.);
#4262=ORIENTED_EDGE('',*,*,#3291,.T.);
#4263=ORIENTED_EDGE('',*,*,#3292,.T.);
#4264=ORIENTED_EDGE('',*,*,#3293,.T.);
#4265=ORIENTED_EDGE('',*,*,#3294,.T.);
#4266=ORIENTED_EDGE('',*,*,#3295,.T.);
#4267=ORIENTED_EDGE('',*,*,#3296,.T.);
#4268=ORIENTED_EDGE('',*,*,#3289,.T.);
#4269=ORIENTED_EDGE('',*,*,#3297,.T.);
#4270=ORIENTED_EDGE('',*,*,#3293,.F.);
#4271=ORIENTED_EDGE('',*,*,#3298,.T.);
#4272=ORIENTED_EDGE('',*,*,#3299,.F.);
#4273=ORIENTED_EDGE('',*,*,#3281,.F.);
#4274=ORIENTED_EDGE('',*,*,#3300,.F.);
#4275=ORIENTED_EDGE('',*,*,#3295,.F.);
#4276=ORIENTED_EDGE('',*,*,#3300,.T.);
#4277=ORIENTED_EDGE('',*,*,#3280,.F.);
#4278=ORIENTED_EDGE('',*,*,#3301,.F.);
#4279=ORIENTED_EDGE('',*,*,#3290,.F.);
#4280=ORIENTED_EDGE('',*,*,#3297,.F.);
#4281=ORIENTED_EDGE('',*,*,#3296,.F.);
#4282=ORIENTED_EDGE('',*,*,#3298,.F.);
#4283=ORIENTED_EDGE('',*,*,#3292,.F.);
#4284=ORIENTED_EDGE('',*,*,#3302,.F.);
#4285=ORIENTED_EDGE('',*,*,#3282,.F.);
#4286=ORIENTED_EDGE('',*,*,#3299,.T.);
#4287=ORIENTED_EDGE('',*,*,#3294,.F.);
#4288=ORIENTED_EDGE('',*,*,#3301,.T.);
#4289=ORIENTED_EDGE('',*,*,#3279,.F.);
#4290=ORIENTED_EDGE('',*,*,#3302,.T.);
#4291=ORIENTED_EDGE('',*,*,#3291,.F.);
#4292=ORIENTED_EDGE('',*,*,#3303,.F.);
#4293=ORIENTED_EDGE('',*,*,#3304,.T.);
#4294=ORIENTED_EDGE('',*,*,#3305,.T.);
#4295=ORIENTED_EDGE('',*,*,#3306,.T.);
#4296=ORIENTED_EDGE('',*,*,#3307,.T.);
#4297=ORIENTED_EDGE('',*,*,#3308,.T.);
#4298=ORIENTED_EDGE('',*,*,#3309,.T.);
#4299=ORIENTED_EDGE('',*,*,#3310,.T.);
#4300=ORIENTED_EDGE('',*,*,#3303,.T.);
#4301=ORIENTED_EDGE('',*,*,#3311,.T.);
#4302=ORIENTED_EDGE('',*,*,#3307,.F.);
#4303=ORIENTED_EDGE('',*,*,#3312,.T.);
#4304=ORIENTED_EDGE('',*,*,#3313,.F.);
#4305=ORIENTED_EDGE('',*,*,#3314,.T.);
#4306=ORIENTED_EDGE('',*,*,#3315,.T.);
#4307=ORIENTED_EDGE('',*,*,#3316,.T.);
#4308=ORIENTED_EDGE('',*,*,#3317,.T.);
#4309=ORIENTED_EDGE('',*,*,#3318,.T.);
#4310=ORIENTED_EDGE('',*,*,#3319,.T.);
#4311=ORIENTED_EDGE('',*,*,#3320,.T.);
#4312=ORIENTED_EDGE('',*,*,#3313,.T.);
#4313=ORIENTED_EDGE('',*,*,#3321,.T.);
#4314=ORIENTED_EDGE('',*,*,#3317,.F.);
#4315=ORIENTED_EDGE('',*,*,#3322,.T.);
#4316=ORIENTED_EDGE('',*,*,#3323,.F.);
#4317=ORIENTED_EDGE('',*,*,#3324,.T.);
#4318=ORIENTED_EDGE('',*,*,#3325,.T.);
#4319=ORIENTED_EDGE('',*,*,#3326,.T.);
#4320=ORIENTED_EDGE('',*,*,#3327,.T.);
#4321=ORIENTED_EDGE('',*,*,#3328,.T.);
#4322=ORIENTED_EDGE('',*,*,#3329,.T.);
#4323=ORIENTED_EDGE('',*,*,#3330,.T.);
#4324=ORIENTED_EDGE('',*,*,#3323,.T.);
#4325=ORIENTED_EDGE('',*,*,#3331,.T.);
#4326=ORIENTED_EDGE('',*,*,#3327,.F.);
#4327=ORIENTED_EDGE('',*,*,#3332,.T.);
#4328=ORIENTED_EDGE('',*,*,#3333,.F.);
#4329=ORIENTED_EDGE('',*,*,#3277,.F.);
#4330=ORIENTED_EDGE('',*,*,#3334,.F.);
#4331=ORIENTED_EDGE('',*,*,#3329,.F.);
#4332=ORIENTED_EDGE('',*,*,#3334,.T.);
#4333=ORIENTED_EDGE('',*,*,#3276,.F.);
#4334=ORIENTED_EDGE('',*,*,#3335,.F.);
#4335=ORIENTED_EDGE('',*,*,#3324,.F.);
#4336=ORIENTED_EDGE('',*,*,#3331,.F.);
#4337=ORIENTED_EDGE('',*,*,#3330,.F.);
#4338=ORIENTED_EDGE('',*,*,#3332,.F.);
#4339=ORIENTED_EDGE('',*,*,#3326,.F.);
#4340=ORIENTED_EDGE('',*,*,#3336,.F.);
#4341=ORIENTED_EDGE('',*,*,#3278,.F.);
#4342=ORIENTED_EDGE('',*,*,#3333,.T.);
#4343=ORIENTED_EDGE('',*,*,#3328,.F.);
#4344=ORIENTED_EDGE('',*,*,#3335,.T.);
#4345=ORIENTED_EDGE('',*,*,#3275,.F.);
#4346=ORIENTED_EDGE('',*,*,#3336,.T.);
#4347=ORIENTED_EDGE('',*,*,#3325,.F.);
#4348=ORIENTED_EDGE('',*,*,#3337,.F.);
#4349=ORIENTED_EDGE('',*,*,#3273,.F.);
#4350=ORIENTED_EDGE('',*,*,#3338,.F.);
#4351=ORIENTED_EDGE('',*,*,#3319,.F.);
#4352=ORIENTED_EDGE('',*,*,#3338,.T.);
#4353=ORIENTED_EDGE('',*,*,#3272,.F.);
#4354=ORIENTED_EDGE('',*,*,#3339,.F.);
#4355=ORIENTED_EDGE('',*,*,#3314,.F.);
#4356=ORIENTED_EDGE('',*,*,#3321,.F.);
#4357=ORIENTED_EDGE('',*,*,#3320,.F.);
#4358=ORIENTED_EDGE('',*,*,#3322,.F.);
#4359=ORIENTED_EDGE('',*,*,#3316,.F.);
#4360=ORIENTED_EDGE('',*,*,#3340,.F.);
#4361=ORIENTED_EDGE('',*,*,#3274,.F.);
#4362=ORIENTED_EDGE('',*,*,#3337,.T.);
#4363=ORIENTED_EDGE('',*,*,#3318,.F.);
#4364=ORIENTED_EDGE('',*,*,#3339,.T.);
#4365=ORIENTED_EDGE('',*,*,#3271,.F.);
#4366=ORIENTED_EDGE('',*,*,#3340,.T.);
#4367=ORIENTED_EDGE('',*,*,#3315,.F.);
#4368=ORIENTED_EDGE('',*,*,#3341,.F.);
#4369=ORIENTED_EDGE('',*,*,#3269,.F.);
#4370=ORIENTED_EDGE('',*,*,#3342,.F.);
#4371=ORIENTED_EDGE('',*,*,#3309,.F.);
#4372=ORIENTED_EDGE('',*,*,#3342,.T.);
#4373=ORIENTED_EDGE('',*,*,#3268,.F.);
#4374=ORIENTED_EDGE('',*,*,#3343,.F.);
#4375=ORIENTED_EDGE('',*,*,#3304,.F.);
#4376=ORIENTED_EDGE('',*,*,#3311,.F.);
#4377=ORIENTED_EDGE('',*,*,#3310,.F.);
#4378=ORIENTED_EDGE('',*,*,#3312,.F.);
#4379=ORIENTED_EDGE('',*,*,#3306,.F.);
#4380=ORIENTED_EDGE('',*,*,#3344,.F.);
#4381=ORIENTED_EDGE('',*,*,#3270,.F.);
#4382=ORIENTED_EDGE('',*,*,#3341,.T.);
#4383=ORIENTED_EDGE('',*,*,#3308,.F.);
#4384=ORIENTED_EDGE('',*,*,#3343,.T.);
#4385=ORIENTED_EDGE('',*,*,#3267,.F.);
#4386=ORIENTED_EDGE('',*,*,#3344,.T.);
#4387=ORIENTED_EDGE('',*,*,#3305,.F.);
#4388=ORIENTED_EDGE('',*,*,#3258,.F.);
#4389=ORIENTED_EDGE('',*,*,#3259,.F.);
#4390=ORIENTED_EDGE('',*,*,#3345,.T.);
#4391=ORIENTED_EDGE('',*,*,#3287,.F.);
#4392=ORIENTED_EDGE('',*,*,#3345,.F.);
#4393=ORIENTED_EDGE('',*,*,#3286,.F.);
#4394=ORIENTED_EDGE('',*,*,#3346,.T.);
#4395=ORIENTED_EDGE('',*,*,#3264,.F.);
#4396=ORIENTED_EDGE('',*,*,#3265,.F.);
#4397=ORIENTED_EDGE('',*,*,#3346,.F.);
#4398=ORIENTED_EDGE('',*,*,#3288,.T.);
#4399=ORIENTED_EDGE('',*,*,#3347,.T.);
#4400=ORIENTED_EDGE('',*,*,#3348,.F.);
#4401=ORIENTED_EDGE('',*,*,#3347,.F.);
#4402=ORIENTED_EDGE('',*,*,#3348,.T.);
#5646=PLANE('',#6352);
#5647=PLANE('',#6354);
#5648=PLANE('',#6360);
#5649=PLANE('',#6362);
#5650=PLANE('',#6371);
#5651=PLANE('',#6373);
#5652=PLANE('',#6378);
#5653=PLANE('',#6380);
#5654=PLANE('',#6385);
#5655=PLANE('',#6387);
#5656=PLANE('',#6407);
#5832=ADVANCED_FACE('',(#783,#646,#647,#648,#649,#650,#651,#652),#499,.T.);
#5833=ADVANCED_FACE('',(#784),#5646,.T.);
#5834=ADVANCED_FACE('',(#785,#653),#5647,.F.);
#5835=ADVANCED_FACE('',(#786),#219,.T.);
#5836=ADVANCED_FACE('',(#787),#220,.T.);
#5837=ADVANCED_FACE('',(#788),#221,.T.);
#5838=ADVANCED_FACE('',(#789),#222,.T.);
#5839=ADVANCED_FACE('',(#790),#500,.T.);
#5840=ADVANCED_FACE('',(#791),#5648,.T.);
#5841=ADVANCED_FACE('',(#792),#5649,.F.);
#5842=ADVANCED_FACE('',(#793),#501,.F.);
#5843=ADVANCED_FACE('',(#794),#199,.F.);
#5844=ADVANCED_FACE('',(#795),#200,.F.);
#5845=ADVANCED_FACE('',(#796),#502,.F.);
#5846=ADVANCED_FACE('',(#797),#503,.T.);
#5847=ADVANCED_FACE('',(#798),#5650,.T.);
#5848=ADVANCED_FACE('',(#799),#5651,.F.);
#5849=ADVANCED_FACE('',(#800),#504,.T.);
#5850=ADVANCED_FACE('',(#801),#5652,.T.);
#5851=ADVANCED_FACE('',(#802),#5653,.F.);
#5852=ADVANCED_FACE('',(#803),#505,.T.);
#5853=ADVANCED_FACE('',(#804),#5654,.T.);
#5854=ADVANCED_FACE('',(#805),#5655,.F.);
#5855=ADVANCED_FACE('',(#806),#506,.F.);
#5856=ADVANCED_FACE('',(#807),#201,.F.);
#5857=ADVANCED_FACE('',(#808),#202,.F.);
#5858=ADVANCED_FACE('',(#809),#507,.F.);
#5859=ADVANCED_FACE('',(#810),#508,.F.);
#5860=ADVANCED_FACE('',(#811),#203,.F.);
#5861=ADVANCED_FACE('',(#812),#204,.F.);
#5862=ADVANCED_FACE('',(#813),#509,.F.);
#5863=ADVANCED_FACE('',(#814),#510,.F.);
#5864=ADVANCED_FACE('',(#815),#205,.F.);
#5865=ADVANCED_FACE('',(#816),#206,.F.);
#5866=ADVANCED_FACE('',(#817),#511,.F.);
#5867=ADVANCED_FACE('',(#818),#207,.T.);
#5868=ADVANCED_FACE('',(#819),#208,.T.);
#5869=ADVANCED_FACE('',(#820),#512,.F.);
#5870=ADVANCED_FACE('',(#821),#5656,.T.);
#6135=CLOSED_SHELL('',(#5832,#5833,#5834,#5835,#5836,#5837,#5838,#5839,
#5840,#5841,#5842,#5843,#5844,#5845,#5846,#5847,#5848,#5849,#5850,#5851,
#5852,#5853,#5854,#5855,#5856,#5857,#5858,#5859,#5860,#5861,#5862,#5863,
#5864,#5865,#5866,#5867,#5868,#5869,#5870));
#6338=AXIS2_PLACEMENT_3D('',#10190,#7133,#7134);
#6339=AXIS2_PLACEMENT_3D('',#10191,#7135,#7136);
#6340=AXIS2_PLACEMENT_3D('',#10194,#7137,#7138);
#6341=AXIS2_PLACEMENT_3D('',#10195,#7139,#7140);
#6342=AXIS2_PLACEMENT_3D('',#10233,#7143,#7144);
#6343=AXIS2_PLACEMENT_3D('',#10234,#7145,#7146);
#6344=AXIS2_PLACEMENT_3D('',#10264,#7148,#7149);
#6345=AXIS2_PLACEMENT_3D('',#10267,#7151,#7152);
#6346=AXIS2_PLACEMENT_3D('',#10272,#7154,#7155);
#6347=AXIS2_PLACEMENT_3D('',#10275,#7157,#7158);
#6348=AXIS2_PLACEMENT_3D('',#10280,#7160,#7161);
#6349=AXIS2_PLACEMENT_3D('',#10283,#7163,#7164);
#6350=AXIS2_PLACEMENT_3D('',#10288,#7166,#7167);
#6351=AXIS2_PLACEMENT_3D('',#10291,#7169,#7170);
#6352=AXIS2_PLACEMENT_3D('',#10427,#7171,#7172);
#6353=AXIS2_PLACEMENT_3D('',#10429,#7173,#7174);
#6354=AXIS2_PLACEMENT_3D('',#10430,#7175,#7176);
#6355=AXIS2_PLACEMENT_3D('',#10432,#7177,#7178);
#6356=AXIS2_PLACEMENT_3D('',#10434,#7179,#7180);
#6357=AXIS2_PLACEMENT_3D('',#10495,#7181,#7182);
#6358=AXIS2_PLACEMENT_3D('',#10498,#7183,#7184);
#6359=AXIS2_PLACEMENT_3D('',#10516,#7186,#7187);
#6360=AXIS2_PLACEMENT_3D('',#10532,#7189,#7190);
#6361=AXIS2_PLACEMENT_3D('',#10533,#7191,#7192);
#6362=AXIS2_PLACEMENT_3D('',#10534,#7193,#7194);
#6363=AXIS2_PLACEMENT_3D('',#10535,#7195,#7196);
#6364=AXIS2_PLACEMENT_3D('',#10536,#7197,#7198);
#6365=AXIS2_PLACEMENT_3D('',#10557,#7199,#7200);
#6366=AXIS2_PLACEMENT_3D('',#10568,#7201,#7202);
#6367=AXIS2_PLACEMENT_3D('',#10579,#7203,#7204);
#6368=AXIS2_PLACEMENT_3D('',#10580,#7205,#7206);
#6369=AXIS2_PLACEMENT_3D('',#10583,#7207,#7208);
#6370=AXIS2_PLACEMENT_3D('',#10601,#7210,#7211);
#6371=AXIS2_PLACEMENT_3D('',#10617,#7213,#7214);
#6372=AXIS2_PLACEMENT_3D('',#10618,#7215,#7216);
#6373=AXIS2_PLACEMENT_3D('',#10619,#7217,#7218);
#6374=AXIS2_PLACEMENT_3D('',#10620,#7219,#7220);
#6375=AXIS2_PLACEMENT_3D('',#10621,#7221,#7222);
#6376=AXIS2_PLACEMENT_3D('',#10624,#7223,#7224);
#6377=AXIS2_PLACEMENT_3D('',#10642,#7226,#7227);
#6378=AXIS2_PLACEMENT_3D('',#10658,#7229,#7230);
#6379=AXIS2_PLACEMENT_3D('',#10659,#7231,#7232);
#6380=AXIS2_PLACEMENT_3D('',#10660,#7233,#7234);
#6381=AXIS2_PLACEMENT_3D('',#10661,#7235,#7236);
#6382=AXIS2_PLACEMENT_3D('',#10662,#7237,#7238);
#6383=AXIS2_PLACEMENT_3D('',#10665,#7239,#7240);
#6384=AXIS2_PLACEMENT_3D('',#10683,#7242,#7243);
#6385=AXIS2_PLACEMENT_3D('',#10699,#7245,#7246);
#6386=AXIS2_PLACEMENT_3D('',#10700,#7247,#7248);
#6387=AXIS2_PLACEMENT_3D('',#10701,#7249,#7250);
#6388=AXIS2_PLACEMENT_3D('',#10702,#7251,#7252);
#6389=AXIS2_PLACEMENT_3D('',#10703,#7253,#7254);
#6390=AXIS2_PLACEMENT_3D('',#10724,#7255,#7256);
#6391=AXIS2_PLACEMENT_3D('',#10735,#7257,#7258);
#6392=AXIS2_PLACEMENT_3D('',#10746,#7259,#7260);
#6393=AXIS2_PLACEMENT_3D('',#10747,#7261,#7262);
#6394=AXIS2_PLACEMENT_3D('',#10768,#7263,#7264);
#6395=AXIS2_PLACEMENT_3D('',#10779,#7265,#7266);
#6396=AXIS2_PLACEMENT_3D('',#10790,#7267,#7268);
#6397=AXIS2_PLACEMENT_3D('',#10791,#7269,#7270);
#6398=AXIS2_PLACEMENT_3D('',#10812,#7271,#7272);
#6399=AXIS2_PLACEMENT_3D('',#10823,#7273,#7274);
#6400=AXIS2_PLACEMENT_3D('',#10834,#7275,#7276);
#6401=AXIS2_PLACEMENT_3D('',#10835,#7277,#7278);
#6402=AXIS2_PLACEMENT_3D('',#10836,#7279,#7280);
#6403=AXIS2_PLACEMENT_3D('',#10837,#7281,#7282);
#6404=AXIS2_PLACEMENT_3D('',#10838,#7283,#7284);
#6405=AXIS2_PLACEMENT_3D('',#10839,#7285,#7286);
#6406=AXIS2_PLACEMENT_3D('',#10842,#7288,#7289);
#6407=AXIS2_PLACEMENT_3D('',#10843,#7290,#7291);
#7133=DIRECTION('axis',(0.,0.,1.));
#7134=DIRECTION('refdir',(1.,0.,0.));
#7135=DIRECTION('center_axis',(-1.,-1.4811191380744E-16,-1.85154420029064E-16));
#7136=DIRECTION('ref_axis',(-1.85154420029064E-16,0.,1.));
#7137=DIRECTION('center_axis',(1.,1.4811191380744E-16,1.85154420029064E-16));
#7138=DIRECTION('ref_axis',(1.85154420029064E-16,0.,-1.));
#7139=DIRECTION('center_axis',(1.,1.4811191380744E-16,1.85154420029064E-16));
#7140=DIRECTION('ref_axis',(1.85154420029064E-16,0.,-1.));
#7141=DIRECTION('',(1.,1.4811191380744E-16,1.85154420029064E-16));
#7142=DIRECTION('',(1.,1.4811191380744E-16,1.85154420029064E-16));
#7143=DIRECTION('center_axis',(1.,1.4811191380744E-16,1.85154420029064E-16));
#7144=DIRECTION('ref_axis',(1.85154420029064E-16,0.,-1.));
#7145=DIRECTION('center_axis',(1.,1.4811191380744E-16,1.85154420029064E-16));
#7146=DIRECTION('ref_axis',(1.85154420029064E-16,0.,-1.));
#7147=DIRECTION('',(-1.,0.,-1.85037170770859E-16));
#7148=DIRECTION('center_axis',(1.,3.00568153244441E-16,7.87229747683671E-17));
#7149=DIRECTION('ref_axis',(-3.00568153244441E-16,1.,0.));
#7150=DIRECTION('',(-1.,0.,-1.96601993944038E-16));
#7151=DIRECTION('center_axis',(1.,3.00568153244441E-16,7.87229747683671E-17));
#7152=DIRECTION('ref_axis',(-3.00568153244441E-16,1.,0.));
#7153=DIRECTION('',(-1.,0.,0.));
#7154=DIRECTION('center_axis',(1.,4.06999598505139E-16,2.3117921420537E-16));
#7155=DIRECTION('ref_axis',(-4.06999598505139E-16,1.,0.));
#7156=DIRECTION('',(-1.,0.,0.));
#7157=DIRECTION('center_axis',(1.,4.06999598505139E-16,2.3117921420537E-16));
#7158=DIRECTION('ref_axis',(-4.06999598505139E-16,1.,0.));
#7159=DIRECTION('',(-1.,0.,-3.70074341541719E-16));
#7160=DIRECTION('center_axis',(1.,2.54543359068137E-16,3.37610659466067E-16));
#7161=DIRECTION('ref_axis',(3.37610659466067E-16,0.,-1.));
#7162=DIRECTION('',(-1.,0.,-3.70074341541719E-16));
#7163=DIRECTION('center_axis',(1.,2.54543359068137E-16,3.37610659466067E-16));
#7164=DIRECTION('ref_axis',(3.37610659466067E-16,0.,-1.));
#7165=DIRECTION('',(-1.,0.,-1.96601993944038E-16));
#7166=DIRECTION('center_axis',(1.,1.4811191380744E-16,1.85154420029064E-16));
#7167=DIRECTION('ref_axis',(1.85154420029064E-16,0.,-1.));
#7168=DIRECTION('',(-1.,0.,-1.38777878078144E-16));
#7169=DIRECTION('center_axis',(1.,1.4811191380744E-16,1.85154420029064E-16));
#7170=DIRECTION('ref_axis',(1.85154420029064E-16,0.,-1.));
#7171=DIRECTION('center_axis',(1.,1.4811191380744E-16,1.85154420029064E-16));
#7172=DIRECTION('ref_axis',(1.85154420029064E-16,0.,-1.));
#7173=DIRECTION('center_axis',(1.,1.4811191380744E-16,1.85154420029064E-16));
#7174=DIRECTION('ref_axis',(1.85154420029064E-16,0.,-1.));
#7175=DIRECTION('center_axis',(1.,1.4811191380744E-16,1.85154420029064E-16));
#7176=DIRECTION('ref_axis',(1.85154420029064E-16,0.,-1.));
#7177=DIRECTION('center_axis',(1.,1.4811191380744E-16,1.85154420029064E-16));
#7178=DIRECTION('ref_axis',(1.85154420029064E-16,0.,-1.));
#7179=DIRECTION('center_axis',(1.,1.4811191380744E-16,1.85154420029064E-16));
#7180=DIRECTION('ref_axis',(1.85154420029064E-16,0.,-1.));
#7181=DIRECTION('center_axis',(-1.,-1.4811191380744E-16,-1.85154420029064E-16));
#7182=DIRECTION('ref_axis',(-1.85154420029064E-16,0.,1.));
#7183=DIRECTION('center_axis',(1.,1.4811191380744E-16,1.85154420029064E-16));
#7184=DIRECTION('ref_axis',(1.85154420029064E-16,0.,-1.));
#7185=DIRECTION('',(-1.,0.,-1.92827419455378E-16));
#7186=DIRECTION('center_axis',(1.,1.4811191380744E-16,1.85154420029064E-16));
#7187=DIRECTION('ref_axis',(1.85154420029064E-16,0.,-1.));
#7188=DIRECTION('',(-1.,0.,-1.65280645247467E-16));
#7189=DIRECTION('center_axis',(1.,1.4811191380744E-16,1.85154420029064E-16));
#7190=DIRECTION('ref_axis',(1.85154420029064E-16,0.,-1.));
#7191=DIRECTION('center_axis',(1.,1.4811191380744E-16,1.85154420029064E-16));
#7192=DIRECTION('ref_axis',(1.85154420029064E-16,0.,-1.));
#7193=DIRECTION('center_axis',(1.,1.4811191380744E-16,1.85154420029064E-16));
#7194=DIRECTION('ref_axis',(1.85154420029064E-16,0.,-1.));
#7195=DIRECTION('center_axis',(1.,1.4811191380744E-16,1.85154420029064E-16));
#7196=DIRECTION('ref_axis',(1.85154420029064E-16,0.,-1.));
#7197=DIRECTION('center_axis',(1.,1.4811191380744E-16,1.85154420029064E-16));
#7198=DIRECTION('ref_axis',(1.85154420029064E-16,0.,-1.));
#7199=DIRECTION('center_axis',(1.,1.4811191380744E-16,1.85154420029064E-16));
#7200=DIRECTION('ref_axis',(3.15796771448933E-16,0.,-1.));
#7201=DIRECTION('center_axis',(1.,1.4811191380744E-16,1.85154420029064E-16));
#7202=DIRECTION('ref_axis',(3.15796771448933E-16,0.,-1.));
#7203=DIRECTION('center_axis',(1.,1.4811191380744E-16,1.85154420029064E-16));
#7204=DIRECTION('ref_axis',(1.85154420029064E-16,0.,-1.));
#7205=DIRECTION('center_axis',(-1.,-3.00568153244441E-16,-7.87229747683671E-17));
#7206=DIRECTION('ref_axis',(3.00568153244441E-16,-1.,0.));
#7207=DIRECTION('center_axis',(1.,3.00568153244441E-16,7.87229747683671E-17));
#7208=DIRECTION('ref_axis',(-3.0056815324444E-16,1.,-1.04744440165294E-14));
#7209=DIRECTION('',(-1.,0.,-5.50935484158224E-17));
#7210=DIRECTION('center_axis',(1.,3.00568153244441E-16,7.87229747683671E-17));
#7211=DIRECTION('ref_axis',(-3.0056815324444E-16,1.,-1.04744440165294E-14));
#7212=DIRECTION('',(-1.,0.,-8.26403226237337E-17));
#7213=DIRECTION('center_axis',(1.,3.00568153244441E-16,7.87229747683671E-17));
#7214=DIRECTION('ref_axis',(7.87229747683671E-17,0.,-1.));
#7215=DIRECTION('center_axis',(1.,3.00568153244441E-16,7.87229747683671E-17));
#7216=DIRECTION('ref_axis',(-3.00568153244441E-16,1.,0.));
#7217=DIRECTION('center_axis',(1.,3.00568153244441E-16,7.87229747683671E-17));
#7218=DIRECTION('ref_axis',(7.87229747683671E-17,0.,-1.));
#7219=DIRECTION('center_axis',(1.,3.00568153244441E-16,7.87229747683671E-17));
#7220=DIRECTION('ref_axis',(-3.00568153244441E-16,1.,0.));
#7221=DIRECTION('center_axis',(-1.,-4.06999598505139E-16,-2.3117921420537E-16));
#7222=DIRECTION('ref_axis',(4.06999598505139E-16,-1.,0.));
#7223=DIRECTION('center_axis',(1.,4.06999598505139E-16,2.3117921420537E-16));
#7224=DIRECTION('ref_axis',(-2.3117921420537E-16,-1.27744465495421E-32,
1.));
#7225=DIRECTION('',(-1.,-4.4074838732658E-16,-4.4074838732658E-16));
#7226=DIRECTION('center_axis',(1.,4.06999598505139E-16,2.3117921420537E-16));
#7227=DIRECTION('ref_axis',(-2.3117921420537E-16,-1.27744465495421E-32,
1.));
#7228=DIRECTION('',(-1.,-8.81496774653158E-16,-4.40748387326579E-16));
#7229=DIRECTION('center_axis',(1.,4.06999598505139E-16,2.3117921420537E-16));
#7230=DIRECTION('ref_axis',(2.3117921420537E-16,0.,-1.));
#7231=DIRECTION('center_axis',(1.,4.06999598505139E-16,2.3117921420537E-16));
#7232=DIRECTION('ref_axis',(-4.06999598505139E-16,1.,0.));
#7233=DIRECTION('center_axis',(1.,4.06999598505139E-16,2.3117921420537E-16));
#7234=DIRECTION('ref_axis',(2.3117921420537E-16,0.,-1.));
#7235=DIRECTION('center_axis',(1.,4.06999598505139E-16,2.3117921420537E-16));
#7236=DIRECTION('ref_axis',(-4.06999598505139E-16,1.,0.));
#7237=DIRECTION('center_axis',(-1.,-2.54543359068137E-16,-3.37610659466067E-16));
#7238=DIRECTION('ref_axis',(5.87374514062376E-17,0.707106781186545,-0.70710678118655));
#7239=DIRECTION('center_axis',(1.,2.54543359068137E-16,3.37610659466067E-16));
#7240=DIRECTION('ref_axis',(2.54543359068136E-16,-1.,3.49148133884313E-15));
#7241=DIRECTION('',(-1.,0.,0.));
#7242=DIRECTION('center_axis',(1.,2.54543359068137E-16,3.37610659466067E-16));
#7243=DIRECTION('ref_axis',(2.54543359068136E-16,-1.,3.49148133884313E-15));
#7244=DIRECTION('',(-1.,0.,-4.40748387326579E-16));
#7245=DIRECTION('center_axis',(1.,2.54543359068137E-16,3.37610659466067E-16));
#7246=DIRECTION('ref_axis',(3.37610659466067E-16,0.,-1.));
#7247=DIRECTION('center_axis',(1.,2.54543359068137E-16,3.37610659466067E-16));
#7248=DIRECTION('ref_axis',(3.37610659466067E-16,0.,-1.));
#7249=DIRECTION('center_axis',(1.,2.54543359068137E-16,3.37610659466067E-16));
#7250=DIRECTION('ref_axis',(3.37610659466067E-16,0.,-1.));
#7251=DIRECTION('center_axis',(1.,2.54543359068137E-16,3.37610659466067E-16));
#7252=DIRECTION('ref_axis',(3.37610659466067E-16,0.,-1.));
#7253=DIRECTION('center_axis',(1.,1.4811191380744E-16,1.85154420029064E-16));
#7254=DIRECTION('ref_axis',(1.85154420029064E-16,0.,-1.));
#7255=DIRECTION('center_axis',(1.,2.54543359068137E-16,3.37610659466067E-16));
#7256=DIRECTION('ref_axis',(3.15796771448933E-16,0.,-1.));
#7257=DIRECTION('center_axis',(1.,2.54543359068137E-16,3.37610659466067E-16));
#7258=DIRECTION('ref_axis',(3.15796771448933E-16,0.,-1.));
#7259=DIRECTION('center_axis',(1.,2.54543359068137E-16,3.37610659466067E-16));
#7260=DIRECTION('ref_axis',(-3.22551558256129E-16,-0.0570045103629633,0.99837392083241));
#7261=DIRECTION('center_axis',(1.,1.4811191380744E-16,1.85154420029064E-16));
#7262=DIRECTION('ref_axis',(-1.93296391409384E-16,0.0570045103629774,0.998373920832409));
#7263=DIRECTION('center_axis',(1.,4.06999598505139E-16,2.3117921420537E-16));
#7264=DIRECTION('ref_axis',(3.15796771448933E-16,0.,-1.));
#7265=DIRECTION('center_axis',(1.,4.06999598505139E-16,2.3117921420537E-16));
#7266=DIRECTION('ref_axis',(3.15796771448933E-16,0.,-1.));
#7267=DIRECTION('center_axis',(1.,4.06999598505139E-16,2.3117921420537E-16));
#7268=DIRECTION('ref_axis',(-4.06999598505139E-16,1.,0.));
#7269=DIRECTION('center_axis',(1.,1.4811191380744E-16,1.85154420029064E-16));
#7270=DIRECTION('ref_axis',(1.85154420029064E-16,0.,-1.));
#7271=DIRECTION('center_axis',(1.,3.00568153244441E-16,7.87229747683671E-17));
#7272=DIRECTION('ref_axis',(0.,0.,-1.));
#7273=DIRECTION('center_axis',(1.,3.00568153244441E-16,7.87229747683671E-17));
#7274=DIRECTION('ref_axis',(0.,0.,-1.));
#7275=DIRECTION('center_axis',(1.,3.00568153244441E-16,7.87229747683671E-17));
#7276=DIRECTION('ref_axis',(-3.00568153244441E-16,1.,0.));
#7277=DIRECTION('center_axis',(1.,1.4811191380744E-16,1.85154420029064E-16));
#7278=DIRECTION('ref_axis',(3.46606212565903E-16,0.,-1.));
#7279=DIRECTION('center_axis',(1.4811191380744E-16,-1.,3.20853184254275E-32));
#7280=DIRECTION('ref_axis',(-2.16628882853689E-16,0.,1.));
#7281=DIRECTION('center_axis',(1.,1.4811191380744E-16,1.85154420029064E-16));
#7282=DIRECTION('ref_axis',(3.46606212565902E-16,0.,-1.));
#7283=DIRECTION('center_axis',(1.4811191380744E-16,-1.,0.));
#7284=DIRECTION('ref_axis',(0.,0.,1.));
#7285=DIRECTION('center_axis',(1.,1.4811191380744E-16,1.85154420029064E-16));
#7286=DIRECTION('ref_axis',(1.85154420029064E-16,0.,-1.));
#7287=DIRECTION('',(1.,1.4811191380744E-16,1.85154420029064E-16));
#7288=DIRECTION('center_axis',(-1.,-1.4811191380744E-16,-1.85154420029064E-16));
#7289=DIRECTION('ref_axis',(-1.85154420029064E-16,0.,1.));
#7290=DIRECTION('center_axis',(-1.,-1.4811191380744E-16,-1.85154420029064E-16));
#7291=DIRECTION('ref_axis',(-1.85154420029064E-16,0.,1.));
#10190=CARTESIAN_POINT('',(0.,0.,0.));
#10191=CARTESIAN_POINT('Origin',(50.,54.6122755947453,-11.9999999999999));
#10192=CARTESIAN_POINT('',(36.,54.6122755947453,-32.4999999999999));
#10193=CARTESIAN_POINT('',(36.,54.6122755947453,8.50000000000008));
#10194=CARTESIAN_POINT('Origin',(36.,54.6122755947453,-11.9999999999999));
#10195=CARTESIAN_POINT('Origin',(36.,54.6122755947453,-11.9999999999999));
#10196=CARTESIAN_POINT('',(36.603289189263,54.6122755947453,-32.4999999999999));
#10197=CARTESIAN_POINT('',(50.,54.6122755947453,-32.4999999999999));
#10198=CARTESIAN_POINT('',(36.7497490222913,54.2658144588871,-32.4970721002132));
#10199=CARTESIAN_POINT('Ctrl Pts',(36.7497490222914,54.2658144588871,-32.4970721002132));
#10200=CARTESIAN_POINT('Ctrl Pts',(36.7079677621958,54.3157388332819,-32.4979159697851));
#10201=CARTESIAN_POINT('Ctrl Pts',(36.6713203406449,54.3700115492414,-32.4986487617911));
#10202=CARTESIAN_POINT('Ctrl Pts',(36.6219970312668,54.4788517884076,-32.4996303938589));
#10203=CARTESIAN_POINT('Ctrl Pts',(36.6075439138862,54.5320464525539,-32.4999158675413));
#10204=CARTESIAN_POINT('Ctrl Pts',(36.6035546196614,54.5952824394035,-32.4999947523746));
#10205=CARTESIAN_POINT('Ctrl Pts',(36.6032891892631,54.6038064661215,-32.4999999999999));
#10206=CARTESIAN_POINT('Ctrl Pts',(36.6032891892631,54.6122755947453,-32.4999999999999));
#10207=CARTESIAN_POINT('',(48.396710810737,54.6122755947453,-32.4999999999999));
#10208=CARTESIAN_POINT('Ctrl Pts',(48.396710810737,54.6122755947453,-32.4999999999999));
#10209=CARTESIAN_POINT('Ctrl Pts',(48.396710810737,54.5998907719614,-32.4999999999999));
#10210=CARTESIAN_POINT('Ctrl Pts',(48.3961431217452,54.5874935361619,-32.4999887774468));
#10211=CARTESIAN_POINT('Ctrl Pts',(48.3891968128691,54.5117737928711,-32.4998514003519));
#10212=CARTESIAN_POINT('Ctrl Pts',(48.3690498018801,54.4529115279532,-32.4994531179785));
#10213=CARTESIAN_POINT('Ctrl Pts',(48.2945766533058,54.3105701888654,-32.49796779174));
#10214=CARTESIAN_POINT('Ctrl Pts',(48.224634010684,54.229506699135,-32.4965615873769));
#10215=CARTESIAN_POINT('Ctrl Pts',(47.9894682579553,54.0138621012104,-32.4917505532513));
#10216=CARTESIAN_POINT('Ctrl Pts',(47.790194476128,53.8921934273276,-32.4875698440548));
#10217=CARTESIAN_POINT('Ctrl Pts',(47.2591893370102,53.6095844257818,-32.4763245946928));
#10218=CARTESIAN_POINT('Ctrl Pts',(46.8036941106391,53.4296399345416,-32.4664417842137));
#10219=CARTESIAN_POINT('Ctrl Pts',(44.8908589619487,52.8583430003526,-32.4291083452159));
#10220=CARTESIAN_POINT('Ctrl Pts',(43.0234357271856,52.6236088262441,-32.4042961436254));
#10221=CARTESIAN_POINT('Ctrl Pts',(39.8390803845175,52.9459866017737,-32.4325402594283));
#10222=CARTESIAN_POINT('Ctrl Pts',(38.8321900018614,53.205505452804,-32.4535208321079));
#10223=CARTESIAN_POINT('Ctrl Pts',(37.7302514044692,53.6201478825653,-32.476460031332));
#10224=CARTESIAN_POINT('Ctrl Pts',(37.4193174431745,53.768280734008,-32.483158770581));
#10225=CARTESIAN_POINT('Ctrl Pts',(37.0379364071817,54.0043124559943,-32.4911694687953));
#10226=CARTESIAN_POINT('Ctrl Pts',(36.8894774405333,54.1120017210872,-32.4942401368472));
#10227=CARTESIAN_POINT('Ctrl Pts',(36.7699059821373,54.2423162108141,-32.4966645914004));
#10228=CARTESIAN_POINT('Ctrl Pts',(36.7596837012345,54.25394352369,-32.4968714463016));
#10229=CARTESIAN_POINT('Ctrl Pts',(36.7497490222914,54.2658144588871,-32.4970721002132));
#10230=CARTESIAN_POINT('',(49.,54.6122755947453,-32.4999999999999));
#10231=CARTESIAN_POINT('',(50.,54.6122755947453,-32.4999999999999));
#10232=CARTESIAN_POINT('',(49.,54.6122755947453,8.50000000000009));
#10233=CARTESIAN_POINT('Origin',(49.,54.6122755947453,-11.9999999999999));
#10234=CARTESIAN_POINT('Origin',(49.,54.6122755947453,-11.9999999999999));
#10235=CARTESIAN_POINT('Ctrl Pts',(36.603289189263,54.6122755947453,-32.4999999999999));
#10236=CARTESIAN_POINT('Ctrl Pts',(36.603289189263,54.6608249084485,-32.4999999999999));
#10237=CARTESIAN_POINT('Ctrl Pts',(36.6119924398781,54.7075701848921,-32.4998281802077));
#10238=CARTESIAN_POINT('Ctrl Pts',(36.6545156775753,54.8307810795885,-32.4989841905835));
#10239=CARTESIAN_POINT('Ctrl Pts',(36.7008380045797,54.9008048487387,-32.4980603157128));
#10240=CARTESIAN_POINT('Ctrl Pts',(36.8625317111402,55.0923640981108,-32.4947934283504));
#10241=CARTESIAN_POINT('Ctrl Pts',(37.0198338309866,55.2093236387767,-32.4915503477017));
#10242=CARTESIAN_POINT('Ctrl Pts',(37.4320685633155,55.4637121723344,-32.482889935361));
#10243=CARTESIAN_POINT('Ctrl Pts',(37.7488381293379,55.611880231403,-32.4760684685696));
#10244=CARTESIAN_POINT('Ctrl Pts',(39.1601676320809,56.1410407225304,-32.4467069002989));
#10245=CARTESIAN_POINT('Ctrl Pts',(40.717083195287,56.4741768433207,-32.4152718262714));
#10246=CARTESIAN_POINT('Ctrl Pts',(42.5,56.4741768433207,-32.4152718262714));
#10247=CARTESIAN_POINT('Ctrl Pts',(43.4574590376155,56.4741768433207,-32.4152718262714));
#10248=CARTESIAN_POINT('Ctrl Pts',(44.4269153217986,56.3794041517536,-32.4246324531227));
#10249=CARTESIAN_POINT('Ctrl Pts',(46.1871857836264,56.0096519365651,-32.4530673729712));
#10250=CARTESIAN_POINT('Ctrl Pts',(46.8757138664064,55.7779082090869,-32.4681777143441));
#10251=CARTESIAN_POINT('Ctrl Pts',(47.6009912659702,55.4395958991355,-32.4835638316369));
#10252=CARTESIAN_POINT('Ctrl Pts',(47.8399918525533,55.309998820274,-32.4886343233478));
#10253=CARTESIAN_POINT('Ctrl Pts',(48.1243771925797,55.091934993814,-32.4945190874943));
#10254=CARTESIAN_POINT('Ctrl Pts',(48.2195690308988,55.0050263124739,-32.4964575266732));
#10255=CARTESIAN_POINT('Ctrl Pts',(48.3274797628088,54.8557541081654,-32.4986259493983));
#10256=CARTESIAN_POINT('Ctrl Pts',(48.3595242538026,54.796889883988,-32.4992631372541));
#10257=CARTESIAN_POINT('Ctrl Pts',(48.3905089403897,54.6939813738137,-32.4998775530034));
#10258=CARTESIAN_POINT('Ctrl Pts',(48.396710810737,54.6531962409273,-32.4999999999999));
#10259=CARTESIAN_POINT('Ctrl Pts',(48.396710810737,54.6122755947453,-32.4999999999999));
#10260=CARTESIAN_POINT('',(36.5,41.5141044679107,3.76984188672031));
#10261=CARTESIAN_POINT('',(48.5,41.5141044679107,3.76984188672031));
#10262=CARTESIAN_POINT('',(48.5,41.5141044679107,3.76984188672031));
#10263=CARTESIAN_POINT('',(48.5,38.8424337080254,1.09817112683513));
#10264=CARTESIAN_POINT('Origin',(48.5,54.6122755947453,-11.9999999999999));
#10265=CARTESIAN_POINT('',(36.5,38.8424337080254,1.09817112683513));
#10266=CARTESIAN_POINT('',(48.5,38.8424337080254,1.09817112683513));
#10267=CARTESIAN_POINT('Origin',(36.5,54.6122755947453,-11.9999999999999));
#10268=CARTESIAN_POINT('',(36.5,38.8424337080252,-25.0981711268347));
#10269=CARTESIAN_POINT('',(48.5,38.8424337080252,-25.0981711268347));
#10270=CARTESIAN_POINT('',(48.5,38.8424337080252,-25.0981711268347));
#10271=CARTESIAN_POINT('',(48.5,41.5141044679105,-27.7698418867199));
#10272=CARTESIAN_POINT('Origin',(48.5,54.6122755947453,-11.9999999999999));
#10273=CARTESIAN_POINT('',(36.5,41.5141044679105,-27.7698418867199));
#10274=CARTESIAN_POINT('',(48.5,41.5141044679105,-27.7698418867199));
#10275=CARTESIAN_POINT('Origin',(36.5,54.6122755947453,-11.9999999999999));
#10276=CARTESIAN_POINT('',(36.5,67.7104467215801,-27.7698418867201));
#10277=CARTESIAN_POINT('',(48.5,67.7104467215801,-27.7698418867201));
#10278=CARTESIAN_POINT('',(48.5,67.7104467215801,-27.7698418867201));
#10279=CARTESIAN_POINT('',(48.5,70.3821174814653,-25.0981711268349));
#10280=CARTESIAN_POINT('Origin',(48.5,54.6122755947453,-11.9999999999999));
#10281=CARTESIAN_POINT('',(36.5,70.3821174814653,-25.0981711268349));
#10282=CARTESIAN_POINT('',(48.5,70.3821174814653,-25.0981711268349));
#10283=CARTESIAN_POINT('Origin',(36.5,54.6122755947453,-11.9999999999999));
#10284=CARTESIAN_POINT('',(36.5,70.3821174814654,1.09817112683487));
#10285=CARTESIAN_POINT('',(48.5,70.3821174814654,1.09817112683488));
#10286=CARTESIAN_POINT('',(48.5,70.3821174814654,1.09817112683488));
#10287=CARTESIAN_POINT('',(48.5,67.7104467215802,3.76984188672011));
#10288=CARTESIAN_POINT('Origin',(48.5,54.6122755947453,-11.9999999999999));
#10289=CARTESIAN_POINT('',(36.5,67.7104467215802,3.76984188672011));
#10290=CARTESIAN_POINT('',(48.5,67.7104467215802,3.76984188672011));
#10291=CARTESIAN_POINT('Origin',(36.5,54.6122755947453,-11.9999999999999));
#10292=CARTESIAN_POINT('',(36.7497652551312,75.1093469933142,-12.3464475251848));
#10293=CARTESIAN_POINT('Ctrl Pts',(42.5,75.0275474210168,-13.8619012485751));
#10294=CARTESIAN_POINT('Ctrl Pts',(41.5425409623847,75.0275474210168,-13.8619012485751));
#10295=CARTESIAN_POINT('Ctrl Pts',(40.5730846782014,75.0369080478681,-13.767128557008));
#10296=CARTESIAN_POINT('Ctrl Pts',(38.8128142163727,75.0653429677166,-13.3973763418193));
#10297=CARTESIAN_POINT('Ctrl Pts',(38.124286133593,75.0804533090896,-13.165632614341));
#10298=CARTESIAN_POINT('Ctrl Pts',(37.39900873403,75.0958394263824,-12.82732030439));
#10299=CARTESIAN_POINT('Ctrl Pts',(37.1600081474468,75.1009099180932,-12.6977232255284));
#10300=CARTESIAN_POINT('Ctrl Pts',(36.8756228074202,75.1067946822398,-12.4796593990683));
#10301=CARTESIAN_POINT('Ctrl Pts',(36.7804309691012,75.1087331214186,-12.3927507177283));
#10302=CARTESIAN_POINT('Ctrl Pts',(36.6725202371911,75.1109015441437,-12.2434785134197));
#10303=CARTESIAN_POINT('Ctrl Pts',(36.6404757461974,75.1115387319995,-12.1846142892423));
#10304=CARTESIAN_POINT('Ctrl Pts',(36.60578337376,75.1122266698925,-12.0693915532655));
#10305=CARTESIAN_POINT('Ctrl Pts',(36.6000950949635,75.1123387689502,-12.0162240743446));
#10306=CARTESIAN_POINT('Ctrl Pts',(36.6108031871309,75.1121269950974,-11.8994981981255));
#10307=CARTESIAN_POINT('Ctrl Pts',(36.63095019812,75.1117287127239,-11.8406359332075));
#10308=CARTESIAN_POINT('Ctrl Pts',(36.705423346694,75.1102433864854,-11.6982945941202));
#10309=CARTESIAN_POINT('Ctrl Pts',(36.7753659893155,75.1088371821223,-11.6172311043898));
#10310=CARTESIAN_POINT('Ctrl Pts',(37.0105317420447,75.1040261479967,-11.4015865064648));
#10311=CARTESIAN_POINT('Ctrl Pts',(37.2098055238719,75.0998454388001,-11.279917832582));
#10312=CARTESIAN_POINT('Ctrl Pts',(37.7408106629901,75.0886001894382,-10.997308831036));
#10313=CARTESIAN_POINT('Ctrl Pts',(38.1963058893614,75.0787173789591,-10.8173643397959));
#10314=CARTESIAN_POINT('Ctrl Pts',(40.1091410380511,75.0413839399612,-10.2460674056071));
#10315=CARTESIAN_POINT('Ctrl Pts',(41.9765642728142,75.0165717383708,-10.0113332314985));
#10316=CARTESIAN_POINT('Ctrl Pts',(45.1609196154824,75.0448158541737,-10.3337110070281));
#10317=CARTESIAN_POINT('Ctrl Pts',(46.1678099981386,75.0657964268533,-10.5932298580583));
#10318=CARTESIAN_POINT('Ctrl Pts',(47.2697485955313,75.0887356260774,-11.0078722878199));
#10319=CARTESIAN_POINT('Ctrl Pts',(47.5806825568259,75.0954343653265,-11.1560051392625));
#10320=CARTESIAN_POINT('Ctrl Pts',(47.9620635928186,75.1034450635407,-11.3920368612488));
#10321=CARTESIAN_POINT('Ctrl Pts',(48.1105225594667,75.1065157315926,-11.4997261263416));
#10322=CARTESIAN_POINT('Ctrl Pts',(48.2739688645561,75.10982980122,-11.6778574474043));
#10323=CARTESIAN_POINT('Ctrl Pts',(48.3224965288387,75.1108012999275,-11.7440918293815));
#10324=CARTESIAN_POINT('Ctrl Pts',(48.3780029687331,75.1119059886043,-11.8665761936618));
#10325=CARTESIAN_POINT('Ctrl Pts',(48.3924560861139,75.1121914622867,-11.9197708578082));
#10326=CARTESIAN_POINT('Ctrl Pts',(48.3995482155258,75.1123317029947,-12.0321911950802));
#10327=CARTESIAN_POINT('Ctrl Pts',(48.3907243897671,75.112157697847,-12.0874225881673));
#10328=CARTESIAN_POINT('Ctrl Pts',(48.3454843224248,75.111259785329,-12.2185054848428));
#10329=CARTESIAN_POINT('Ctrl Pts',(48.2991619954204,75.1103359104582,-12.2885292539931));
#10330=CARTESIAN_POINT('Ctrl Pts',(48.1374682888594,75.1070690230958,-12.4800885033658));
#10331=CARTESIAN_POINT('Ctrl Pts',(47.9801661690123,75.1038259424471,-12.5970480440319));
#10332=CARTESIAN_POINT('Ctrl Pts',(47.567931436684,75.0951655301064,-12.8514365775891));
#10333=CARTESIAN_POINT('Ctrl Pts',(47.2511618706613,75.088344063315,-12.9996046366577));
#10334=CARTESIAN_POINT('Ctrl Pts',(45.8398323679192,75.0589824950443,-13.5287651277848));
#10335=CARTESIAN_POINT('Ctrl Pts',(44.2829168047132,75.0275474210168,-13.8619012485751));
#10336=CARTESIAN_POINT('Ctrl Pts',(42.5,75.0275474210168,-13.8619012485751));
#10337=CARTESIAN_POINT('',(36.7497162970046,54.2657870626157,8.49707235020499));
#10338=CARTESIAN_POINT('Ctrl Pts',(42.5,56.4741768433204,8.41527182627157));
#10339=CARTESIAN_POINT('Ctrl Pts',(41.5425409623847,56.4741768433204,8.41527182627157));
#10340=CARTESIAN_POINT('Ctrl Pts',(40.5730846782016,56.3794041517534,8.42463245312286));
#10341=CARTESIAN_POINT('Ctrl Pts',(38.8128142163725,56.0096519365646,8.45306737297136));
#10342=CARTESIAN_POINT('Ctrl Pts',(38.1242861335929,55.7779082090862,8.46817771434433));
#10343=CARTESIAN_POINT('Ctrl Pts',(37.3990087340298,55.4395958991352,8.48356383163711));
#10344=CARTESIAN_POINT('Ctrl Pts',(37.1600081474467,55.3099988202737,8.48863432334797));
#10345=CARTESIAN_POINT('Ctrl Pts',(36.8756228074202,55.0919349938136,8.49451908749452));
#10346=CARTESIAN_POINT('Ctrl Pts',(36.7804309691012,55.0050263124736,8.49645752667339));
#10347=CARTESIAN_POINT('Ctrl Pts',(36.6725202371913,54.8557541081652,8.49862594939842));
#10348=CARTESIAN_POINT('Ctrl Pts',(36.6404757461974,54.7968898839877,8.49926313725424));
#10349=CARTESIAN_POINT('Ctrl Pts',(36.60578337376,54.6816671480108,8.4999510751473));
#10350=CARTESIAN_POINT('Ctrl Pts',(36.6000950949635,54.6284996690899,8.50006317420492));
#10351=CARTESIAN_POINT('Ctrl Pts',(36.6108031871309,54.5117737928708,8.4998514003521));
#10352=CARTESIAN_POINT('Ctrl Pts',(36.63095019812,54.4529115279528,8.49945311797868));
#10353=CARTESIAN_POINT('Ctrl Pts',(36.7054233466942,54.3105701888652,8.49796779174013));
#10354=CARTESIAN_POINT('Ctrl Pts',(36.7753659893159,54.2295066991348,8.49656158737708));
#10355=CARTESIAN_POINT('Ctrl Pts',(37.0105317420448,54.01386210121,8.49175055325143));
#10356=CARTESIAN_POINT('Ctrl Pts',(37.2098055238722,53.8921934273273,8.48756984405489));
#10357=CARTESIAN_POINT('Ctrl Pts',(37.7408106629893,53.6095844257818,8.47632459469298));
#10358=CARTESIAN_POINT('Ctrl Pts',(38.1963058893602,53.4296399345416,8.46644178421388));
#10359=CARTESIAN_POINT('Ctrl Pts',(40.1091410380517,52.8583430003522,8.42910834521598));
#10360=CARTESIAN_POINT('Ctrl Pts',(41.9765642728151,52.623608826244,8.40429614362558));
#10361=CARTESIAN_POINT('Ctrl Pts',(45.1609196154835,52.9459866017735,8.43254025942847));
#10362=CARTESIAN_POINT('Ctrl Pts',(46.1678099981393,53.2055054528039,8.45352083210801));
#10363=CARTESIAN_POINT('Ctrl Pts',(47.2697485955285,53.6201478825642,8.47646003133207));
#10364=CARTESIAN_POINT('Ctrl Pts',(47.5806825568242,53.7682807340069,8.48315877058117));
#10365=CARTESIAN_POINT('Ctrl Pts',(47.9620635928186,54.0043124559941,8.49116946879544));
#10366=CARTESIAN_POINT('Ctrl Pts',(48.1105225594668,54.112001721087,8.49424013684733));
#10367=CARTESIAN_POINT('Ctrl Pts',(48.2739688645561,54.2901330421496,8.49755420647477));
#10368=CARTESIAN_POINT('Ctrl Pts',(48.3224965288387,54.3563674241268,8.49852570518227));
#10369=CARTESIAN_POINT('Ctrl Pts',(48.3780029687332,54.4788517884074,8.49963039385909));
#10370=CARTESIAN_POINT('Ctrl Pts',(48.3924560861139,54.5320464525537,8.49991586754141));
#10371=CARTESIAN_POINT('Ctrl Pts',(48.3995482155258,54.6444667898256,8.50005610824948));
#10372=CARTESIAN_POINT('Ctrl Pts',(48.390724389767,54.6996981829127,8.49988210310169));
#10373=CARTESIAN_POINT('Ctrl Pts',(48.3454843224248,54.8307810795882,8.49898419058371));
#10374=CARTESIAN_POINT('Ctrl Pts',(48.2991619954204,54.9008048487383,8.498060315713));
#10375=CARTESIAN_POINT('Ctrl Pts',(48.13746828886,55.0923640981104,8.49479342835062));
#10376=CARTESIAN_POINT('Ctrl Pts',(47.9801661690137,55.2093236387763,8.49155034770193));
#10377=CARTESIAN_POINT('Ctrl Pts',(47.5679314366844,55.4637121723342,8.48288993536117));
#10378=CARTESIAN_POINT('Ctrl Pts',(47.251161870662,55.6118802314028,8.47606846856981));
#10379=CARTESIAN_POINT('Ctrl Pts',(45.8398323679184,56.1410407225304,8.4467069002991));
#10380=CARTESIAN_POINT('Ctrl Pts',(44.2829168047119,56.4741768433204,8.41527182627157));
#10381=CARTESIAN_POINT('Ctrl Pts',(42.5,56.4741768433204,8.41527182627157));
#10382=CARTESIAN_POINT('',(36.7497162970046,34.1152032445404,-12.3464885321295));
#10383=CARTESIAN_POINT('Ctrl Pts',(42.5,34.1970037684738,-10.1380987514247));
#10384=CARTESIAN_POINT('Ctrl Pts',(41.5425409623847,34.1970037684738,-10.1380987514247));
#10385=CARTESIAN_POINT('Ctrl Pts',(40.5730846782015,34.1876431416225,-10.2328714429918));
#10386=CARTESIAN_POINT('Ctrl Pts',(38.8128142163735,34.1592082217741,-10.6026236581803));
#10387=CARTESIAN_POINT('Ctrl Pts',(38.1242861335935,34.1440978804011,-10.8343673856586));
#10388=CARTESIAN_POINT('Ctrl Pts',(37.39900873403,34.1287117631083,-11.1726796956099));
#10389=CARTESIAN_POINT('Ctrl Pts',(37.1600081474469,34.1236412713974,-11.3022767744714));
#10390=CARTESIAN_POINT('Ctrl Pts',(36.8756228074203,34.1177565072509,-11.5203406009315));
#10391=CARTESIAN_POINT('Ctrl Pts',(36.7804309691013,34.115818068072,-11.6072492822715));
#10392=CARTESIAN_POINT('Ctrl Pts',(36.6725202371913,34.113649645347,-11.75652148658));
#10393=CARTESIAN_POINT('Ctrl Pts',(36.6404757461974,34.1130124574912,-11.8153857107575));
#10394=CARTESIAN_POINT('Ctrl Pts',(36.60578337376,34.1123245195981,-11.9306084467343));
#10395=CARTESIAN_POINT('Ctrl Pts',(36.6000950949635,34.1122124205405,-11.9837759256552));
#10396=CARTESIAN_POINT('Ctrl Pts',(36.6108031871309,34.1124241943933,-12.1005018018743));
#10397=CARTESIAN_POINT('Ctrl Pts',(36.63095019812,34.1128224767667,-12.1593640667924));
#10398=CARTESIAN_POINT('Ctrl Pts',(36.7054233466949,34.1143078030053,-12.3017054058813));
#10399=CARTESIAN_POINT('Ctrl Pts',(36.7753659893176,34.1157140073684,-12.3827688956119));
#10400=CARTESIAN_POINT('Ctrl Pts',(37.0105317420447,34.120525041494,-12.598413493535));
#10401=CARTESIAN_POINT('Ctrl Pts',(37.2098055238719,34.1247057506905,-12.7200821674178));
#10402=CARTESIAN_POINT('Ctrl Pts',(37.7408106629894,34.1359510000524,-13.0026911689634));
#10403=CARTESIAN_POINT('Ctrl Pts',(38.1963058893603,34.1458338105315,-13.1826356602036));
#10404=CARTESIAN_POINT('Ctrl Pts',(40.1091410380501,34.1831672495294,-13.7539325943925));
#10405=CARTESIAN_POINT('Ctrl Pts',(41.9765642728128,34.2079794511198,-13.9886667685015));
#10406=CARTESIAN_POINT('Ctrl Pts',(45.160919615482,34.1797353353169,-13.6662889929718));
#10407=CARTESIAN_POINT('Ctrl Pts',(46.1678099981384,34.1587547626374,-13.4067701419416));
#10408=CARTESIAN_POINT('Ctrl Pts',(47.2697485955313,34.1358155634133,-12.99212771218));
#10409=CARTESIAN_POINT('Ctrl Pts',(47.5806825568258,34.1291168241642,-12.8439948607373));
#10410=CARTESIAN_POINT('Ctrl Pts',(47.9620635928185,34.12110612595,-12.6079631387512));
#10411=CARTESIAN_POINT('Ctrl Pts',(48.1105225594667,34.1180354578981,-12.5002738736583));
#10412=CARTESIAN_POINT('Ctrl Pts',(48.273968864556,34.1147213882706,-12.3221425525957));
#10413=CARTESIAN_POINT('Ctrl Pts',(48.3224965288387,34.1137498895631,-12.2559081706184));
#10414=CARTESIAN_POINT('Ctrl Pts',(48.3780029687333,34.1126452008863,-12.1334238063378));
#10415=CARTESIAN_POINT('Ctrl Pts',(48.3924560861139,34.112359727204,-12.0802291421916));
#10416=CARTESIAN_POINT('Ctrl Pts',(48.3995482155258,34.1122194864959,-11.9678088049197));
#10417=CARTESIAN_POINT('Ctrl Pts',(48.3907243897671,34.1123934916437,-11.9125774118326));
#10418=CARTESIAN_POINT('Ctrl Pts',(48.3454843224248,34.1132914041617,-11.7814945151571));
#10419=CARTESIAN_POINT('Ctrl Pts',(48.2991619954205,34.1142152790324,-11.7114707460069));
#10420=CARTESIAN_POINT('Ctrl Pts',(48.1374682888603,34.1174821663948,-11.5199114966352));
#10421=CARTESIAN_POINT('Ctrl Pts',(47.9801661690144,34.1207252470435,-11.4029519559693));
#10422=CARTESIAN_POINT('Ctrl Pts',(47.5679314366847,34.1293856593842,-11.1485634224112));
#10423=CARTESIAN_POINT('Ctrl Pts',(47.2511618706624,34.1362071261756,-11.0003953633426));
#10424=CARTESIAN_POINT('Ctrl Pts',(45.8398323679199,34.1655686944463,-10.4712348722153));
#10425=CARTESIAN_POINT('Ctrl Pts',(44.2829168047143,34.1970037684738,-10.1380987514247));
#10426=CARTESIAN_POINT('Ctrl Pts',(42.5,34.1970037684738,-10.1380987514247));
#10427=CARTESIAN_POINT('Origin',(50.,54.6122755947453,-11.9999999999999));
#10428=CARTESIAN_POINT('',(50.,54.6122755947453,7.50000000000009));
#10429=CARTESIAN_POINT('Origin',(50.,54.6122755947453,-11.9999999999999));
#10430=CARTESIAN_POINT('Origin',(35.,54.6122755947453,-11.9999999999999));
#10431=CARTESIAN_POINT('',(35.,54.6122755947453,7.50000000000008));
#10432=CARTESIAN_POINT('Origin',(35.,54.6122755947453,-11.9999999999999));
#10433=CARTESIAN_POINT('',(35.,54.6122755947453,5.50000000000008));
#10434=CARTESIAN_POINT('Origin',(35.,54.6122755947453,-11.9999999999999));
#10435=CARTESIAN_POINT('Ctrl Pts',(36.6000954047721,75.6303323723191,-11.0710623055408));
#10436=CARTESIAN_POINT('Ctrl Pts',(36.6000954047721,75.1163129851934,-11.390036451076));
#10437=CARTESIAN_POINT('Ctrl Pts',(36.6000954047721,75.113533389205,-11.9949767040821));
#10438=CARTESIAN_POINT('Ctrl Pts',(36.6000954047721,75.1107537932165,-12.5999169570882));
#10439=CARTESIAN_POINT('Ctrl Pts',(36.6000954047721,75.6218202760576,-12.923601195162));
#10440=CARTESIAN_POINT('Ctrl Pts',(42.4997945641984,74.4160919611753,-9.11434223685902));
#10441=CARTESIAN_POINT('Ctrl Pts',(42.4997945641984,72.8193389779435,-10.1052054829035));
#10442=CARTESIAN_POINT('Ctrl Pts',(42.4997945641984,72.8107044238821,-11.9843956026886));
#10443=CARTESIAN_POINT('Ctrl Pts',(42.4997945641984,72.8020698698207,-13.8635857224736));
#10444=CARTESIAN_POINT('Ctrl Pts',(42.4997945641984,74.3896499330349,-14.8690804289273));
#10445=CARTESIAN_POINT('Ctrl Pts',(48.3995480441881,75.630258991695,-11.0709440543786));
#10446=CARTESIAN_POINT('Ctrl Pts',(48.3995480441881,75.1161741713435,-11.3899588044276));
#10447=CARTESIAN_POINT('Ctrl Pts',(48.3995480441881,75.1133942215203,-11.9949760646306));
#10448=CARTESIAN_POINT('Ctrl Pts',(48.3995480441881,75.1106142716971,-12.5999933248336));
#10449=CARTESIAN_POINT('Ctrl Pts',(48.3995480441881,75.6217458118676,-12.9237187670028));
#10450=CARTESIAN_POINT('Ctrl Pts',(36.6000954047721,53.6833379002862,9.01805677757378));
#10451=CARTESIAN_POINT('Ctrl Pts',(36.6000954047721,54.0023120458214,8.50403739044816));
#10452=CARTESIAN_POINT('Ctrl Pts',(36.6000954047721,54.6072522988275,8.50125779445973));
#10453=CARTESIAN_POINT('Ctrl Pts',(36.6000954047721,55.2121925518336,8.4984781984713));
#10454=CARTESIAN_POINT('Ctrl Pts',(36.6000954047721,55.5358767899073,9.00954468131236));
#10455=CARTESIAN_POINT('Ctrl Pts',(42.4997945641984,51.7266178316045,7.80381636642986));
#10456=CARTESIAN_POINT('Ctrl Pts',(42.4997945641984,52.7174810776491,6.2070633831982));
#10457=CARTESIAN_POINT('Ctrl Pts',(42.4997945641984,54.596671197434,6.19842882913689));
#10458=CARTESIAN_POINT('Ctrl Pts',(42.4997945641984,56.4758613172189,6.18979427507558));
#10459=CARTESIAN_POINT('Ctrl Pts',(42.4997945641984,57.4813560236726,7.77737433828968));
#10460=CARTESIAN_POINT('Ctrl Pts',(48.3995480441881,53.683219649124,9.0179833969497));
#10461=CARTESIAN_POINT('Ctrl Pts',(48.3995480441881,54.002234399173,8.50389857659829));
#10462=CARTESIAN_POINT('Ctrl Pts',(48.3995480441881,54.607251659376,8.50111862677509));
#10463=CARTESIAN_POINT('Ctrl Pts',(48.3995480441881,55.212268919579,8.49833867695189));
#10464=CARTESIAN_POINT('Ctrl Pts',(48.3995480441881,55.5359943617481,9.00947021712231));
#10465=CARTESIAN_POINT('Ctrl Pts',(36.6000954047722,33.5942188171715,-12.9289376944591));
#10466=CARTESIAN_POINT('Ctrl Pts',(36.6000954047722,34.1082382042972,-12.6099635489239));
#10467=CARTESIAN_POINT('Ctrl Pts',(36.6000954047722,34.1110178002857,-12.0050232959178));
#10468=CARTESIAN_POINT('Ctrl Pts',(36.6000954047722,34.1137973962741,-11.4000830429116));
#10469=CARTESIAN_POINT('Ctrl Pts',(36.6000954047722,33.602730913433,-11.0763988048379));
#10470=CARTESIAN_POINT('Ctrl Pts',(42.4997945641985,34.8084592283153,-14.8856577631409));
#10471=CARTESIAN_POINT('Ctrl Pts',(42.4997945641985,36.4052122115471,-13.8947945170964));
#10472=CARTESIAN_POINT('Ctrl Pts',(42.4997945641985,36.4138467656085,-12.0156043973113));
#10473=CARTESIAN_POINT('Ctrl Pts',(42.4997945641985,36.4224813196699,-10.1364142775263));
#10474=CARTESIAN_POINT('Ctrl Pts',(42.4997945641985,34.8349012564557,-9.13091957107256));
#10475=CARTESIAN_POINT('Ctrl Pts',(48.3995480441881,33.5942921977956,-12.9290559456212));
#10476=CARTESIAN_POINT('Ctrl Pts',(48.3995480441881,34.1083770181471,-12.6100411955723));
#10477=CARTESIAN_POINT('Ctrl Pts',(48.3995480441881,34.1111569679703,-12.0050239353692));
#10478=CARTESIAN_POINT('Ctrl Pts',(48.3995480441881,34.1139369177935,-11.4000066751662));
#10479=CARTESIAN_POINT('Ctrl Pts',(48.3995480441881,33.6028053776231,-11.0762812329971));
#10480=CARTESIAN_POINT('Ctrl Pts',(36.603289189263,55.5369296408085,-33.0088778576148));
#10481=CARTESIAN_POINT('Ctrl Pts',(36.603289189263,55.2128764217899,-32.4972287891192));
#10482=CARTESIAN_POINT('Ctrl Pts',(36.603289189263,54.6072465725666,-32.5000115536831));
#10483=CARTESIAN_POINT('Ctrl Pts',(36.603289189263,54.0016167233433,-32.5027943182471));
#10484=CARTESIAN_POINT('Ctrl Pts',(36.603289189263,53.682278966091,-33.0173996571641));
#10485=CARTESIAN_POINT('Ctrl Pts',(42.5,57.4802106040728,-31.7780997904234));
#10486=CARTESIAN_POINT('Ctrl Pts',(42.5,56.4751173200863,-30.1911535349279));
#10487=CARTESIAN_POINT('Ctrl Pts',(42.5,54.5966774271594,-30.1997846418264));
#10488=CARTESIAN_POINT('Ctrl Pts',(42.5,52.7182375342324,-30.2084157487249));
#10489=CARTESIAN_POINT('Ctrl Pts',(42.5,51.7277698693544,-31.8045312621439));
#10490=CARTESIAN_POINT('Ctrl Pts',(48.396710810737,55.5369296408085,-33.0088778576148));
#10491=CARTESIAN_POINT('Ctrl Pts',(48.396710810737,55.2128764217899,-32.4972287891192));
#10492=CARTESIAN_POINT('Ctrl Pts',(48.396710810737,54.6072465725666,-32.5000115536831));
#10493=CARTESIAN_POINT('Ctrl Pts',(48.396710810737,54.0016167233433,-32.5027943182471));
#10494=CARTESIAN_POINT('Ctrl Pts',(48.396710810737,53.682278966091,-33.0173996571641));
#10495=CARTESIAN_POINT('Origin',(47.5,69.4571012113211,2.84482561657582));
#10496=CARTESIAN_POINT('',(47.5,70.4387355541152,2.55242815321436));
#10497=CARTESIAN_POINT('',(47.5,69.1647037479597,3.82645995936986));
#10498=CARTESIAN_POINT('Origin',(47.5,69.4571012113211,2.84482561657582));
#10499=CARTESIAN_POINT('',(47.537899429919,70.3143910047143,2.28432898886365));
#10500=CARTESIAN_POINT('Ctrl Pts',(47.5,70.4387355541152,2.55242815321436));
#10501=CARTESIAN_POINT('Ctrl Pts',(47.5,70.4189527998948,2.48601365455714));
#10502=CARTESIAN_POINT('Ctrl Pts',(47.5053044417601,70.3925771182096,2.422112506851));
#10503=CARTESIAN_POINT('Ctrl Pts',(47.5230476022983,70.3458637388305,2.33479395638985));
#10504=CARTESIAN_POINT('Ctrl Pts',(47.5298073931343,70.3305302530218,2.30901426289197));
#10505=CARTESIAN_POINT('Ctrl Pts',(47.537899429919,70.3143910047143,2.28432898886365));
#10506=CARTESIAN_POINT('',(37.4621005700809,70.3143910047143,2.28432898886365));
#10507=CARTESIAN_POINT('',(47.537899429919,70.3143910047143,2.28432898886365));
#10508=CARTESIAN_POINT('',(37.5,70.4387355541152,2.55242815321436));
#10509=CARTESIAN_POINT('Ctrl Pts',(37.462100570081,70.3143910047143,2.28432898886366));
#10510=CARTESIAN_POINT('Ctrl Pts',(37.4632744099609,70.3167321820717,2.28790986224227));
#10511=CARTESIAN_POINT('Ctrl Pts',(37.4644207388779,70.3190574281895,2.29151535342116));
#10512=CARTESIAN_POINT('Ctrl Pts',(37.4898409184866,70.371513910436,2.37399296978792));
#10513=CARTESIAN_POINT('Ctrl Pts',(37.5,70.4113518729136,2.46049588543571));
#10514=CARTESIAN_POINT('Ctrl Pts',(37.5,70.4387355541152,2.55242815321435));
#10515=CARTESIAN_POINT('',(37.5,69.1647037479597,3.82645995936986));
#10516=CARTESIAN_POINT('Origin',(37.5,69.4571012113211,2.84482561657581));
#10517=CARTESIAN_POINT('',(37.4621005700809,68.8966045836089,3.70211540996904));
#10518=CARTESIAN_POINT('Ctrl Pts',(37.5,69.1647037479597,3.82645995936986));
#10519=CARTESIAN_POINT('Ctrl Pts',(37.5,69.0990912208333,3.80691608680946));
#10520=CARTESIAN_POINT('Ctrl Pts',(37.4948229521317,69.0359160073849,3.78093293985881));
#10521=CARTESIAN_POINT('Ctrl Pts',(37.4773121076774,68.948446705185,3.73440602894735));
#10522=CARTESIAN_POINT('Ctrl Pts',(37.470409170669,68.9219504993238,3.7186865862433));
#10523=CARTESIAN_POINT('Ctrl Pts',(37.462100570081,68.896604583609,3.70211540996904));
#10524=CARTESIAN_POINT('',(47.5378994299191,68.8966045836089,3.70211540996904));
#10525=CARTESIAN_POINT('',(47.5378994299191,68.8966045836089,3.70211540996904));
#10526=CARTESIAN_POINT('Ctrl Pts',(47.537899429919,68.8966045836089,3.70211540996903));
#10527=CARTESIAN_POINT('Ctrl Pts',(47.5369318666484,68.8995561970421,3.7040451767624));
#10528=CARTESIAN_POINT('Ctrl Pts',(47.5359829808858,68.9025245795757,3.7059641473824));
#10529=CARTESIAN_POINT('Ctrl Pts',(47.510332174293,68.9848409778267,3.75857431922063));
#10530=CARTESIAN_POINT('Ctrl Pts',(47.5,69.0719944289914,3.79884481948067));
#10531=CARTESIAN_POINT('Ctrl Pts',(47.5,69.1647037479597,3.82645995936986));
#10532=CARTESIAN_POINT('Origin',(47.5,54.6122755947453,-11.9999999999999));
#10533=CARTESIAN_POINT('Origin',(47.5,54.6122755947453,-11.9999999999999));
#10534=CARTESIAN_POINT('Origin',(37.5,54.6122755947453,-11.9999999999999));
#10535=CARTESIAN_POINT('Origin',(37.5,54.6122755947453,-11.9999999999999));
#10536=CARTESIAN_POINT('Origin',(47.5,68.349381898499,4.5391024665601));
#10537=CARTESIAN_POINT('Ctrl Pts',(37.4621005700809,68.896604583609,3.70211540996902));
#10538=CARTESIAN_POINT('Ctrl Pts',(37.4310083838403,68.8017558875511,3.6401032704416));
#10539=CARTESIAN_POINT('Ctrl Pts',(37.3828779782886,68.7018867262922,3.59772631179564));
#10540=CARTESIAN_POINT('Ctrl Pts',(37.245031822289,68.4694900791145,3.53679150015867));
#10541=CARTESIAN_POINT('Ctrl Pts',(37.1423703640038,68.3305669520952,3.52988534954539));
#10542=CARTESIAN_POINT('Ctrl Pts',(36.8667626334574,68.017493954875,3.57885731564907));
#10543=CARTESIAN_POINT('Ctrl Pts',(36.6872103879512,67.8515747651484,3.65364745765698));
#10544=CARTESIAN_POINT('Ctrl Pts',(36.5029780432796,67.7126857281249,3.76798632698662));
#10545=CARTESIAN_POINT('Ctrl Pts',(36.5014890205786,67.711565210995,3.76891288782061));
#10546=CARTESIAN_POINT('Ctrl Pts',(36.5,67.7104467215802,3.76984188672011));
#10547=CARTESIAN_POINT('Ctrl Pts',(47.537899429919,68.896604583609,3.70211540996901));
#10548=CARTESIAN_POINT('Ctrl Pts',(47.5689916161593,68.8017558875522,3.64010327044235));
#10549=CARTESIAN_POINT('Ctrl Pts',(47.6171220217102,68.7018867262946,3.59772631179665));
#10550=CARTESIAN_POINT('Ctrl Pts',(47.7549681777082,68.4694900791187,3.53679150015924));
#10551=CARTESIAN_POINT('Ctrl Pts',(47.8576296359926,68.3305669520998,3.52988534954533));
#10552=CARTESIAN_POINT('Ctrl Pts',(48.1332373665856,68.0174939548254,3.57885731565596));
#10553=CARTESIAN_POINT('Ctrl Pts',(48.3127896121225,67.8515747651177,3.65364745768193));
#10554=CARTESIAN_POINT('Ctrl Pts',(48.4970219567203,67.7126857281242,3.76798632698724));
#10555=CARTESIAN_POINT('Ctrl Pts',(48.498510979422,67.7115652109945,3.76891288782097));
#10556=CARTESIAN_POINT('Ctrl Pts',(48.5,67.7104467215802,3.7698418867201));
#10557=CARTESIAN_POINT('Origin',(48.5,54.6122755947453,-11.9999999999999));
#10558=CARTESIAN_POINT('Ctrl Pts',(47.537899429919,70.3143910047143,2.28432898886365));
#10559=CARTESIAN_POINT('Ctrl Pts',(47.5689916161588,70.2523788651886,2.18948029280836));
#10560=CARTESIAN_POINT('Ctrl Pts',(47.6171220217088,70.2100019065432,2.08961113155225));
#10561=CARTESIAN_POINT('Ctrl Pts',(47.7549681777051,70.1490670949051,1.85721448437786));
#10562=CARTESIAN_POINT('Ctrl Pts',(47.8576296359887,70.1421609442907,1.71829135735951));
#10563=CARTESIAN_POINT('Ctrl Pts',(48.1332373666213,70.1911329104067,1.40521836003877));
#10564=CARTESIAN_POINT('Ctrl Pts',(48.3127896121854,70.2659230524474,1.23929917034817));
#10565=CARTESIAN_POINT('Ctrl Pts',(48.4970219567186,70.3802619217321,1.10041013337938));
#10566=CARTESIAN_POINT('Ctrl Pts',(48.4985109794219,70.3811884825662,1.09928961624927));
#10567=CARTESIAN_POINT('Ctrl Pts',(48.5,70.3821174814654,1.09817112683487));
#10568=CARTESIAN_POINT('Origin',(36.5,54.6122755947453,-11.9999999999999));
#10569=CARTESIAN_POINT('Ctrl Pts',(37.4621005700809,70.3143910047143,2.28432898886365));
#10570=CARTESIAN_POINT('Ctrl Pts',(37.4310083838412,70.2523788651887,2.18948029280845));
#10571=CARTESIAN_POINT('Ctrl Pts',(37.3828779782913,70.2100019065433,2.08961113155242));
#10572=CARTESIAN_POINT('Ctrl Pts',(37.2450318222954,70.1490670949052,1.85721448437858));
#10573=CARTESIAN_POINT('Ctrl Pts',(37.1423703640119,70.1421609442906,1.71829135736027));
#10574=CARTESIAN_POINT('Ctrl Pts',(36.8667626333773,70.1911329104068,1.40521836003708));
#10575=CARTESIAN_POINT('Ctrl Pts',(36.6872103878129,70.2659230524489,1.23929917034637));
#10576=CARTESIAN_POINT('Ctrl Pts',(36.5029780432807,70.3802619217326,1.10041013337885));
#10577=CARTESIAN_POINT('Ctrl Pts',(36.5014890205792,70.3811884825656,1.09928961625003));
#10578=CARTESIAN_POINT('Ctrl Pts',(36.5,70.3821174814654,1.09817112683487));
#10579=CARTESIAN_POINT('Origin',(50.,71.1513780613054,1.73710630375365));
#10580=CARTESIAN_POINT('Origin',(47.5,39.7674499781698,2.84482561657604));
#10581=CARTESIAN_POINT('',(47.5,40.0598474415312,3.82645995937007));
#10582=CARTESIAN_POINT('',(47.5,38.7858156353757,2.5524281532146));
#10583=CARTESIAN_POINT('Origin',(47.5,39.7674499781698,2.84482561657604));
#10584=CARTESIAN_POINT('',(47.5378994299191,40.3279466058819,3.70211540996925));
#10585=CARTESIAN_POINT('Ctrl Pts',(47.5,40.0598474415312,3.82645995937007));
#10586=CARTESIAN_POINT('Ctrl Pts',(47.5,40.1262619401886,3.80667720514962));
#10587=CARTESIAN_POINT('Ctrl Pts',(47.5053044417602,40.1901630878949,3.7803015234644));
#10588=CARTESIAN_POINT('Ctrl Pts',(47.5230476022984,40.277481638356,3.73358814408523));
#10589=CARTESIAN_POINT('Ctrl Pts',(47.5298073931343,40.3032613318537,3.71825465827663));
#10590=CARTESIAN_POINT('Ctrl Pts',(47.537899429919,40.3279466058819,3.70211540996925));
#10591=CARTESIAN_POINT('',(37.462100570081,40.3279466058819,3.70211540996925));
#10592=CARTESIAN_POINT('',(47.5378994299191,40.3279466058819,3.70211540996925));
#10593=CARTESIAN_POINT('',(37.5,40.0598474415312,3.82645995937007));
#10594=CARTESIAN_POINT('Ctrl Pts',(37.462100570081,40.3279466058819,3.70211540996925));
#10595=CARTESIAN_POINT('Ctrl Pts',(37.4632744099609,40.3243657325033,3.70445658732663));
#10596=CARTESIAN_POINT('Ctrl Pts',(37.4644207388779,40.3207602413243,3.70678183344449));
#10597=CARTESIAN_POINT('Ctrl Pts',(37.4898409184866,40.2382826249574,3.75923831569102));
#10598=CARTESIAN_POINT('Ctrl Pts',(37.5,40.1517797093097,3.7990762781686));
#10599=CARTESIAN_POINT('Ctrl Pts',(37.5,40.0598474415312,3.82645995937007));
#10600=CARTESIAN_POINT('',(37.5,38.7858156353757,2.55242815321459));
#10601=CARTESIAN_POINT('Origin',(37.5,39.7674499781698,2.84482561657603));
#10602=CARTESIAN_POINT('',(37.462100570081,38.9101601847765,2.28432898886388));
#10603=CARTESIAN_POINT('Ctrl Pts',(37.5,38.7858156353757,2.55242815321459));
#10604=CARTESIAN_POINT('Ctrl Pts',(37.5,38.8053595079361,2.48681562608814));
#10605=CARTESIAN_POINT('Ctrl Pts',(37.4948229521316,38.8313426548868,2.42364041263967));
#10606=CARTESIAN_POINT('Ctrl Pts',(37.4773121076774,38.8778695657982,2.33617111043986));
#10607=CARTESIAN_POINT('Ctrl Pts',(37.470409170669,38.8935890085023,2.3096749045787));
#10608=CARTESIAN_POINT('Ctrl Pts',(37.462100570081,38.9101601847765,2.28432898886388));
#10609=CARTESIAN_POINT('',(47.5378994299191,38.9101601847765,2.28432898886388));
#10610=CARTESIAN_POINT('',(47.5378994299191,38.9101601847765,2.28432898886388));
#10611=CARTESIAN_POINT('Ctrl Pts',(47.537899429919,38.9101601847765,2.28432898886389));
#10612=CARTESIAN_POINT('Ctrl Pts',(47.5369318666484,38.9082304179831,2.28728060229702));
#10613=CARTESIAN_POINT('Ctrl Pts',(47.5359829808858,38.9063114473632,2.29024898483066));
#10614=CARTESIAN_POINT('Ctrl Pts',(47.5103321742929,38.8537012755249,2.37256538308168));
#10615=CARTESIAN_POINT('Ctrl Pts',(47.5,38.8134307752649,2.45971883424642));
#10616=CARTESIAN_POINT('Ctrl Pts',(47.5,38.7858156353757,2.5524281532146));
#10617=CARTESIAN_POINT('Origin',(47.5,54.6122755947453,-11.9999999999999));
#10618=CARTESIAN_POINT('Origin',(47.5,54.6122755947453,-11.9999999999999));
#10619=CARTESIAN_POINT('Origin',(37.5,54.6122755947453,-11.9999999999999));
#10620=CARTESIAN_POINT('Origin',(37.5,54.6122755947453,-11.9999999999999));
#10621=CARTESIAN_POINT('Origin',(47.5,39.7674499781695,-26.8448256165756));
#10622=CARTESIAN_POINT('',(47.5,38.7858156353755,-26.5524281532142));
#10623=CARTESIAN_POINT('',(47.5,40.059847441531,-27.8264599593697));
#10624=CARTESIAN_POINT('Origin',(47.5,39.7674499781695,-26.8448256165756));
#10625=CARTESIAN_POINT('',(47.5378994299191,38.9101601847763,-26.2843289888635));
#10626=CARTESIAN_POINT('Ctrl Pts',(47.5,38.7858156353755,-26.5524281532142));
#10627=CARTESIAN_POINT('Ctrl Pts',(47.5,38.8055983895958,-26.4860136545571));
#10628=CARTESIAN_POINT('Ctrl Pts',(47.5053044417601,38.8319740712809,-26.4221125068513));
#10629=CARTESIAN_POINT('Ctrl Pts',(47.5230476022982,38.8786874506599,-26.3347939563902));
#10630=CARTESIAN_POINT('Ctrl Pts',(47.5298073931342,38.8940209364687,-26.309014262892));
#10631=CARTESIAN_POINT('Ctrl Pts',(47.5378994299191,38.9101601847763,-26.2843289888635));
#10632=CARTESIAN_POINT('',(37.462100570081,38.9101601847763,-26.2843289888635));
#10633=CARTESIAN_POINT('',(47.5378994299191,38.9101601847763,-26.2843289888635));
#10634=CARTESIAN_POINT('',(37.5,38.7858156353755,-26.5524281532142));
#10635=CARTESIAN_POINT('Ctrl Pts',(37.462100570081,38.9101601847763,-26.2843289888635));
#10636=CARTESIAN_POINT('Ctrl Pts',(37.463274409961,38.9078190074188,-26.2879098622423));
#10637=CARTESIAN_POINT('Ctrl Pts',(37.464420738878,38.9054937613009,-26.2915153534214));
#10638=CARTESIAN_POINT('Ctrl Pts',(37.4898409184867,38.8530372790542,-26.3739929697886));
#10639=CARTESIAN_POINT('Ctrl Pts',(37.5,38.8131993165768,-26.4604958854362));
#10640=CARTESIAN_POINT('Ctrl Pts',(37.5,38.7858156353755,-26.5524281532142));
#10641=CARTESIAN_POINT('',(37.5,40.059847441531,-27.8264599593697));
#10642=CARTESIAN_POINT('Origin',(37.5,39.7674499781695,-26.8448256165756));
#10643=CARTESIAN_POINT('',(37.462100570081,40.3279466058817,-27.7021154099689));
#10644=CARTESIAN_POINT('Ctrl Pts',(37.5,40.059847441531,-27.8264599593697));
#10645=CARTESIAN_POINT('Ctrl Pts',(37.5,40.1254599686575,-27.8069160868092));
#10646=CARTESIAN_POINT('Ctrl Pts',(37.4948229521316,40.1886351821059,-27.7809329398586));
#10647=CARTESIAN_POINT('Ctrl Pts',(37.4773121076774,40.2761044843057,-27.7344060289472));
#10648=CARTESIAN_POINT('Ctrl Pts',(37.470409170669,40.3026006901669,-27.7186865862431));
#10649=CARTESIAN_POINT('Ctrl Pts',(37.462100570081,40.3279466058817,-27.7021154099689));
#10650=CARTESIAN_POINT('',(47.5378994299191,40.3279466058817,-27.7021154099689));
#10651=CARTESIAN_POINT('',(47.5378994299191,40.3279466058817,-27.7021154099689));
#10652=CARTESIAN_POINT('Ctrl Pts',(47.5378994299191,40.3279466058817,-27.7021154099689));
#10653=CARTESIAN_POINT('Ctrl Pts',(47.5369318666484,40.3249949924486,-27.7040451767622));
#10654=CARTESIAN_POINT('Ctrl Pts',(47.5359829808858,40.3220266099149,-27.7059641473822));
#10655=CARTESIAN_POINT('Ctrl Pts',(47.5103321742929,40.2397102116637,-27.7585743192207));
#10656=CARTESIAN_POINT('Ctrl Pts',(47.5,40.1525567604989,-27.7988448194806));
#10657=CARTESIAN_POINT('Ctrl Pts',(47.5,40.059847441531,-27.8264599593697));
#10658=CARTESIAN_POINT('Origin',(47.5,54.6122755947453,-11.9999999999999));
#10659=CARTESIAN_POINT('Origin',(47.5,54.6122755947453,-11.9999999999999));
#10660=CARTESIAN_POINT('Origin',(37.5,54.6122755947453,-11.9999999999999));
#10661=CARTESIAN_POINT('Origin',(37.5,54.6122755947453,-11.9999999999999));
#10662=CARTESIAN_POINT('Origin',(47.5,69.457101211321,-26.8448256165758));
#10663=CARTESIAN_POINT('',(47.5,69.1647037479595,-27.8264599593698));
#10664=CARTESIAN_POINT('',(47.5,70.4387355541151,-26.5524281532143));
#10665=CARTESIAN_POINT('Origin',(47.5,69.457101211321,-26.8448256165758));
#10666=CARTESIAN_POINT('',(47.5378994299191,68.8966045836088,-27.702115409969));
#10667=CARTESIAN_POINT('Ctrl Pts',(47.5,69.1647037479595,-27.8264599593698));
#10668=CARTESIAN_POINT('Ctrl Pts',(47.5,69.0982892493024,-27.8066772051495));
#10669=CARTESIAN_POINT('Ctrl Pts',(47.5053044417601,69.0343881015963,-27.7803015234644));
#10670=CARTESIAN_POINT('Ctrl Pts',(47.5230476022983,68.9470695511352,-27.7335881440852));
#10671=CARTESIAN_POINT('Ctrl Pts',(47.5298073931342,68.9212898576372,-27.7182546582765));
#10672=CARTESIAN_POINT('Ctrl Pts',(47.5378994299191,68.8966045836088,-27.702115409969));
#10673=CARTESIAN_POINT('',(37.462100570081,68.8966045836088,-27.702115409969));
#10674=CARTESIAN_POINT('',(47.5378994299191,68.8966045836088,-27.702115409969));
#10675=CARTESIAN_POINT('',(37.5,69.1647037479595,-27.8264599593698));
#10676=CARTESIAN_POINT('Ctrl Pts',(37.462100570081,68.8966045836088,-27.702115409969));
#10677=CARTESIAN_POINT('Ctrl Pts',(37.4632744099607,68.900185456987,-27.704456587326));
#10678=CARTESIAN_POINT('Ctrl Pts',(37.4644207388776,68.9037909481654,-27.7067818334436));
#10679=CARTESIAN_POINT('Ctrl Pts',(37.4898409184865,68.9862685645324,-27.7592383156903));
#10680=CARTESIAN_POINT('Ctrl Pts',(37.5,69.0727714801806,-27.7990762781682));
#10681=CARTESIAN_POINT('Ctrl Pts',(37.5,69.1647037479595,-27.8264599593698));
#10682=CARTESIAN_POINT('',(37.5,70.4387355541151,-26.5524281532143));
#10683=CARTESIAN_POINT('Origin',(37.5,69.457101211321,-26.8448256165758));
#10684=CARTESIAN_POINT('',(37.462100570081,70.3143910047142,-26.2843289888636));
#10685=CARTESIAN_POINT('Ctrl Pts',(37.5,70.4387355541151,-26.5524281532143));
#10686=CARTESIAN_POINT('Ctrl Pts',(37.5,70.4191916815546,-26.4868156260878));
#10687=CARTESIAN_POINT('Ctrl Pts',(37.4948229521316,70.3932085346039,-26.4236404126394));
#10688=CARTESIAN_POINT('Ctrl Pts',(37.4773121076774,70.3466816236925,-26.3361711104396));
#10689=CARTESIAN_POINT('Ctrl Pts',(37.470409170669,70.3309621809885,-26.3096749045784));
#10690=CARTESIAN_POINT('Ctrl Pts',(37.462100570081,70.3143910047142,-26.2843289888636));
#10691=CARTESIAN_POINT('',(47.5378994299191,70.3143910047142,-26.2843289888636));
#10692=CARTESIAN_POINT('',(47.5378994299191,70.3143910047142,-26.2843289888636));
#10693=CARTESIAN_POINT('Ctrl Pts',(47.5378994299191,70.3143910047142,-26.2843289888636));
#10694=CARTESIAN_POINT('Ctrl Pts',(47.5369318666484,70.3163207715076,-26.2872806022967));
#10695=CARTESIAN_POINT('Ctrl Pts',(47.5359829808858,70.3182397421275,-26.2902489848303));
#10696=CARTESIAN_POINT('Ctrl Pts',(47.510332174293,70.3708499139657,-26.3725653830812));
#10697=CARTESIAN_POINT('Ctrl Pts',(47.5,70.4111204142258,-26.4597188342459));
#10698=CARTESIAN_POINT('Ctrl Pts',(47.5,70.4387355541151,-26.5524281532143));
#10699=CARTESIAN_POINT('Origin',(47.5,54.6122755947453,-11.9999999999999));
#10700=CARTESIAN_POINT('Origin',(47.5,54.6122755947453,-11.9999999999999));
#10701=CARTESIAN_POINT('Origin',(37.5,54.6122755947453,-11.9999999999999));
#10702=CARTESIAN_POINT('Origin',(37.5,54.6122755947453,-11.9999999999999));
#10703=CARTESIAN_POINT('Origin',(47.5,71.1513780613053,-25.7371063037536));
#10704=CARTESIAN_POINT('Ctrl Pts',(37.462100570081,70.3143910047142,-26.2843289888636));
#10705=CARTESIAN_POINT('Ctrl Pts',(37.4310083838417,70.2523788651895,-26.1894802928099));
#10706=CARTESIAN_POINT('Ctrl Pts',(37.3828779782928,70.2100019065445,-26.0896111315555));
#10707=CARTESIAN_POINT('Ctrl Pts',(37.2450318222992,70.1490670949059,-25.8572144843843));
#10708=CARTESIAN_POINT('Ctrl Pts',(37.1423703640169,70.1421609442904,-25.7182913573665));
#10709=CARTESIAN_POINT('Ctrl Pts',(36.8667626333183,70.1911329104162,-25.4052183599692));
#10710=CARTESIAN_POINT('Ctrl Pts',(36.6872103877121,70.2659230524829,-25.2392991703043));
#10711=CARTESIAN_POINT('Ctrl Pts',(36.5029780432812,70.3802619217331,-25.1004101333781));
#10712=CARTESIAN_POINT('Ctrl Pts',(36.5014890205775,70.3811884825665,-25.0992896162488));
#10713=CARTESIAN_POINT('Ctrl Pts',(36.5,70.3821174814653,-25.0981711268349));
#10714=CARTESIAN_POINT('Ctrl Pts',(47.5378994299191,70.3143910047142,-26.2843289888636));
#10715=CARTESIAN_POINT('Ctrl Pts',(47.568991616158,70.2523788651901,-26.1894802928108));
#10716=CARTESIAN_POINT('Ctrl Pts',(47.6171220217063,70.2100019065453,-26.0896111315574));
#10717=CARTESIAN_POINT('Ctrl Pts',(47.7549681776988,70.1490670949063,-25.8572144843871));
#10718=CARTESIAN_POINT('Ctrl Pts',(47.8576296359807,70.1421609442904,-25.7182913573697));
#10719=CARTESIAN_POINT('Ctrl Pts',(48.1332373667109,70.1911329104208,-25.4052183599355));
#10720=CARTESIAN_POINT('Ctrl Pts',(48.3127896123394,70.2659230524989,-25.2392991702846));
#10721=CARTESIAN_POINT('Ctrl Pts',(48.4970219567185,70.3802619217334,-25.1004101333777));
#10722=CARTESIAN_POINT('Ctrl Pts',(48.4985109794227,70.3811884825666,-25.0992896162486));
#10723=CARTESIAN_POINT('Ctrl Pts',(48.5,70.3821174814653,-25.0981711268349));
#10724=CARTESIAN_POINT('Origin',(48.5,54.6122755947453,-11.9999999999999));
#10725=CARTESIAN_POINT('Ctrl Pts',(47.5378994299191,68.8966045836088,-27.702115409969));
#10726=CARTESIAN_POINT('Ctrl Pts',(47.5689916161593,68.8017558875521,-27.6401032704423));
#10727=CARTESIAN_POINT('Ctrl Pts',(47.6171220217102,68.7018867262945,-27.5977263117966));
#10728=CARTESIAN_POINT('Ctrl Pts',(47.7549681777078,68.4694900791192,-27.5367915001594));
#10729=CARTESIAN_POINT('Ctrl Pts',(47.857629635992,68.3305669521004,-27.5298853495452));
#10730=CARTESIAN_POINT('Ctrl Pts',(48.1332373665661,68.0174939548474,-27.5788573156524));
#10731=CARTESIAN_POINT('Ctrl Pts',(48.3127896120915,67.8515747651331,-27.6536474576698));
#10732=CARTESIAN_POINT('Ctrl Pts',(48.4970219567174,67.7126857281265,-27.7679863269852));
#10733=CARTESIAN_POINT('Ctrl Pts',(48.4985109794222,67.7115652109942,-27.7689128878211));
#10734=CARTESIAN_POINT('Ctrl Pts',(48.5,67.71044672158,-27.7698418867201));
#10735=CARTESIAN_POINT('Origin',(36.5,54.6122755947453,-11.9999999999999));
#10736=CARTESIAN_POINT('Ctrl Pts',(37.462100570081,68.8966045836088,-27.702115409969));
#10737=CARTESIAN_POINT('Ctrl Pts',(37.4310083838413,68.8017558875538,-27.6401032704434));
#10738=CARTESIAN_POINT('Ctrl Pts',(37.3828779782915,68.701886726298,-27.5977263117981));
#10739=CARTESIAN_POINT('Ctrl Pts',(37.245031822296,68.4694900791247,-27.5367915001601));
#10740=CARTESIAN_POINT('Ctrl Pts',(37.1423703640128,68.3305669521065,-27.5298853495452));
#10741=CARTESIAN_POINT('Ctrl Pts',(36.8667626333661,68.0174939547694,-27.5788573156634));
#10742=CARTESIAN_POINT('Ctrl Pts',(36.6872103877933,67.8515747650841,-27.6536474577095));
#10743=CARTESIAN_POINT('Ctrl Pts',(36.5029780432822,67.7126857281249,-27.7679863269865));
#10744=CARTESIAN_POINT('Ctrl Pts',(36.5014890205769,67.7115652109935,-27.7689128878217));
#10745=CARTESIAN_POINT('Ctrl Pts',(36.5,67.71044672158,-27.7698418867201));
#10746=CARTESIAN_POINT('Origin',(50.,68.3493818984988,-28.5391024665601));
#10747=CARTESIAN_POINT('Origin',(47.5,40.8751692909917,-28.5391024665599));
#10748=CARTESIAN_POINT('Ctrl Pts',(37.462100570081,40.3279466058817,-27.7021154099689));
#10749=CARTESIAN_POINT('Ctrl Pts',(37.4310083838416,40.4227953019356,-27.640103270444));
#10750=CARTESIAN_POINT('Ctrl Pts',(37.3828779782926,40.5226644631903,-27.5977263117989));
#10751=CARTESIAN_POINT('Ctrl Pts',(37.2450318222986,40.755061110362,-27.5367915001605));
#10752=CARTESIAN_POINT('Ctrl Pts',(37.1423703640161,40.8939842373798,-27.529885349545));
#10753=CARTESIAN_POINT('Ctrl Pts',(36.8667626333263,41.2070572347668,-27.5788573156696));
#10754=CARTESIAN_POINT('Ctrl Pts',(36.6872103877253,41.3729764244348,-27.6536474577325));
#10755=CARTESIAN_POINT('Ctrl Pts',(36.5029780432813,41.511865461367,-27.7679863269875));
#10756=CARTESIAN_POINT('Ctrl Pts',(36.5014890205774,41.5129859784966,-27.7689128878212));
#10757=CARTESIAN_POINT('Ctrl Pts',(36.5,41.5141044679104,-27.7698418867199));
#10758=CARTESIAN_POINT('Ctrl Pts',(47.5378994299191,40.3279466058817,-27.7021154099689));
#10759=CARTESIAN_POINT('Ctrl Pts',(47.5689916161584,40.4227953019356,-27.640103270444));
#10760=CARTESIAN_POINT('Ctrl Pts',(47.6171220217074,40.5226644631902,-27.597726311799));
#10761=CARTESIAN_POINT('Ctrl Pts',(47.7549681777013,40.7550611103619,-27.5367915001605));
#10762=CARTESIAN_POINT('Ctrl Pts',(47.8576296359839,40.8939842373797,-27.5298853495451));
#10763=CARTESIAN_POINT('Ctrl Pts',(48.1332373666762,41.2070572347697,-27.57885731567));
#10764=CARTESIAN_POINT('Ctrl Pts',(48.3127896122781,41.3729764244373,-27.6536474577346));
#10765=CARTESIAN_POINT('Ctrl Pts',(48.497021956718,41.5118654613665,-27.7679863269871));
#10766=CARTESIAN_POINT('Ctrl Pts',(48.4985109794233,41.5129859784971,-27.7689128878216));
#10767=CARTESIAN_POINT('Ctrl Pts',(48.5,41.5141044679105,-27.7698418867199));
#10768=CARTESIAN_POINT('Origin',(48.5,54.6122755947453,-11.9999999999999));
#10769=CARTESIAN_POINT('Ctrl Pts',(47.5378994299191,38.9101601847763,-26.2843289888635));
#10770=CARTESIAN_POINT('Ctrl Pts',(47.5689916161584,38.9721723243012,-26.1894802928096));
#10771=CARTESIAN_POINT('Ctrl Pts',(47.6171220217074,39.0145492829462,-26.0896111315549));
#10772=CARTESIAN_POINT('Ctrl Pts',(47.7549681777013,39.0754840945847,-25.8572144843834));
#10773=CARTESIAN_POINT('Ctrl Pts',(47.8576296359838,39.0823902452002,-25.7182913573655));
#10774=CARTESIAN_POINT('Ctrl Pts',(48.1332373666738,39.0334182790756,-25.4052183599782));
#10775=CARTESIAN_POINT('Ctrl Pts',(48.3127896122749,38.9586281370126,-25.2392991703103));
#10776=CARTESIAN_POINT('Ctrl Pts',(48.497021956719,38.8442892677574,-25.1004101333779));
#10777=CARTESIAN_POINT('Ctrl Pts',(48.4985109794223,38.8433627069242,-25.0992896162488));
#10778=CARTESIAN_POINT('Ctrl Pts',(48.5,38.8424337080252,-25.0981711268347));
#10779=CARTESIAN_POINT('Origin',(36.5,54.6122755947453,-11.9999999999999));
#10780=CARTESIAN_POINT('Ctrl Pts',(37.462100570081,38.9101601847763,-26.2843289888635));
#10781=CARTESIAN_POINT('Ctrl Pts',(37.4310083838421,38.9721723243003,-26.1894802928109));
#10782=CARTESIAN_POINT('Ctrl Pts',(37.3828779782939,39.0145492829451,-26.0896111315576));
#10783=CARTESIAN_POINT('Ctrl Pts',(37.2450318223019,39.075484094584,-25.8572144843881));
#10784=CARTESIAN_POINT('Ctrl Pts',(37.1423703640203,39.0823902452002,-25.7182913573708));
#10785=CARTESIAN_POINT('Ctrl Pts',(36.8667626332853,39.0334182790692,-25.4052183599309));
#10786=CARTESIAN_POINT('Ctrl Pts',(36.6872103876556,38.9586281369882,-25.2392991702806));
#10787=CARTESIAN_POINT('Ctrl Pts',(36.502978043283,38.844289267758,-25.1004101333787));
#10788=CARTESIAN_POINT('Ctrl Pts',(36.5014890205765,38.8433627069234,-25.0992896162479));
#10789=CARTESIAN_POINT('Ctrl Pts',(36.5,38.8424337080252,-25.0981711268347));
#10790=CARTESIAN_POINT('Origin',(50.,38.0731731281852,-25.7371063037535));
#10791=CARTESIAN_POINT('Origin',(47.5,38.0731731281855,1.73710630375391));
#10792=CARTESIAN_POINT('Ctrl Pts',(37.462100570081,38.9101601847765,2.2843289888639));
#10793=CARTESIAN_POINT('Ctrl Pts',(37.4310083838418,38.9721723243011,2.1894802928104));
#10794=CARTESIAN_POINT('Ctrl Pts',(37.382877978293,39.0145492829461,2.0896111315562));
#10795=CARTESIAN_POINT('Ctrl Pts',(37.2450318222997,39.0754840945847,1.85721448438531));
#10796=CARTESIAN_POINT('Ctrl Pts',(37.1423703640175,39.0823902452004,1.71829135736766));
#10797=CARTESIAN_POINT('Ctrl Pts',(36.8667626333158,39.0334182790742,1.40521835996645));
#10798=CARTESIAN_POINT('Ctrl Pts',(36.6872103877081,38.9586281370059,1.23929917030242));
#10799=CARTESIAN_POINT('Ctrl Pts',(36.5029780432818,38.844289267758,1.10041013337881));
#10800=CARTESIAN_POINT('Ctrl Pts',(36.5014890205776,38.8433627069243,1.09928961624914));
#10801=CARTESIAN_POINT('Ctrl Pts',(36.5,38.8424337080254,1.09817112683512));
#10802=CARTESIAN_POINT('Ctrl Pts',(47.5378994299191,38.9101601847765,2.2843289888639));
#10803=CARTESIAN_POINT('Ctrl Pts',(47.5689916161585,38.9721723243016,2.18948029280961));
#10804=CARTESIAN_POINT('Ctrl Pts',(47.6171220217078,39.0145492829468,2.08961113155459));
#10805=CARTESIAN_POINT('Ctrl Pts',(47.7549681777024,39.0754840945851,1.85721448438222));
#10806=CARTESIAN_POINT('Ctrl Pts',(47.8576296359852,39.0823902452003,1.71829135736426));
#10807=CARTESIAN_POINT('Ctrl Pts',(48.1332373666565,39.0334182790786,1.40521835999846));
#10808=CARTESIAN_POINT('Ctrl Pts',(48.3127896122453,38.9586281370227,1.23929917032299));
#10809=CARTESIAN_POINT('Ctrl Pts',(48.4970219567186,38.8442892677582,1.10041013337901));
#10810=CARTESIAN_POINT('Ctrl Pts',(48.4985109794219,38.8433627069246,1.09928961624948));
#10811=CARTESIAN_POINT('Ctrl Pts',(48.5,38.8424337080254,1.09817112683513));
#10812=CARTESIAN_POINT('Origin',(48.5,54.6122755947453,-11.9999999999999));
#10813=CARTESIAN_POINT('Ctrl Pts',(47.5378994299191,40.3279466058819,3.70211540996925));
#10814=CARTESIAN_POINT('Ctrl Pts',(47.5689916161576,40.4227953019335,3.64010327044594));
#10815=CARTESIAN_POINT('Ctrl Pts',(47.6171220217051,40.5226644631856,3.59772631180138));
#10816=CARTESIAN_POINT('Ctrl Pts',(47.7549681776959,40.7550611103542,3.53679150016188));
#10817=CARTESIAN_POINT('Ctrl Pts',(47.857629635977,40.8939842373711,3.5298853495454));
#10818=CARTESIAN_POINT('Ctrl Pts',(48.1332373667501,41.2070572348553,3.57885731568198));
#10819=CARTESIAN_POINT('Ctrl Pts',(48.3127896124051,41.3729764244901,3.65364745777795));
#10820=CARTESIAN_POINT('Ctrl Pts',(48.4970219567172,41.5118654613675,3.76798632698816));
#10821=CARTESIAN_POINT('Ctrl Pts',(48.4985109794234,41.5129859784975,3.76891288782207));
#10822=CARTESIAN_POINT('Ctrl Pts',(48.5,41.5141044679107,3.76984188672031));
#10823=CARTESIAN_POINT('Origin',(36.5,54.6122755947453,-11.9999999999999));
#10824=CARTESIAN_POINT('Ctrl Pts',(37.462100570081,40.3279466058819,3.70211540996925));
#10825=CARTESIAN_POINT('Ctrl Pts',(37.4310083838421,40.4227953019343,3.64010327044543));
#10826=CARTESIAN_POINT('Ctrl Pts',(37.3828779782942,40.5226644631872,3.5977263118007));
#10827=CARTESIAN_POINT('Ctrl Pts',(37.2450318223022,40.755061110357,3.53679150016149));
#10828=CARTESIAN_POINT('Ctrl Pts',(37.1423703640206,40.8939842373742,3.52988534954544));
#10829=CARTESIAN_POINT('Ctrl Pts',(36.8667626332747,41.2070572348267,3.57885731567809));
#10830=CARTESIAN_POINT('Ctrl Pts',(36.6872103876371,41.3729764244722,3.65364745776331));
#10831=CARTESIAN_POINT('Ctrl Pts',(36.5029780432816,41.511865461368,3.76798632698854));
#10832=CARTESIAN_POINT('Ctrl Pts',(36.5014890205776,41.5129859784967,3.76891288782145));
#10833=CARTESIAN_POINT('Ctrl Pts',(36.5,41.5141044679107,3.76984188672031));
#10834=CARTESIAN_POINT('Origin',(50.,40.8751692909919,4.53910246656033));
#10835=CARTESIAN_POINT('Origin',(36.,54.6122755947453,-11.9999999999999));
#10836=CARTESIAN_POINT('Origin',(36.,54.6122755947453,7.50000000000008));
#10837=CARTESIAN_POINT('Origin',(49.,54.6122755947453,-11.9999999999999));
#10838=CARTESIAN_POINT('Origin',(49.,54.6122755947453,7.50000000000009));
#10839=CARTESIAN_POINT('Origin',(34.999988,54.6122755947453,-11.9999999999999));
#10840=CARTESIAN_POINT('',(45.,54.6122755947453,5.50000000000009));
#10841=CARTESIAN_POINT('',(34.999988,54.6122755947453,5.50000000000008));
#10842=CARTESIAN_POINT('Origin',(45.,54.6122755947453,-11.9999999999999));
#10843=CARTESIAN_POINT('Origin',(45.,54.6122755947453,-11.9999999999999));
#14102=UNCERTAINTY_MEASURE_WITH_UNIT(LENGTH_MEASURE(0.01),#14126,
'DISTANCE_ACCURACY_VALUE',
'Maximum model space distance between geometric entities at asserted c
onnectivities');
#14112=UNCERTAINTY_MEASURE_WITH_UNIT(LENGTH_MEASURE(0.01),#14126,
'DISTANCE_ACCURACY_VALUE',
'Maximum model space distance between geometric entities at asserted c
onnectivities');
#14115=(
GEOMETRIC_REPRESENTATION_CONTEXT(3)
GLOBAL_UNCERTAINTY_ASSIGNED_CONTEXT((#14102))
GLOBAL_UNIT_ASSIGNED_CONTEXT((#14126,#14128,#14129))
REPRESENTATION_CONTEXT('','3D')
);
#14125=(
GEOMETRIC_REPRESENTATION_CONTEXT(3)
GLOBAL_UNCERTAINTY_ASSIGNED_CONTEXT((#14112))
GLOBAL_UNIT_ASSIGNED_CONTEXT((#14126,#14128,#14129))
REPRESENTATION_CONTEXT('','3D')
);
#14126=(
LENGTH_UNIT()
NAMED_UNIT(*)
SI_UNIT(.MILLI.,.METRE.)
);
#14128=(
NAMED_UNIT(*)
PLANE_ANGLE_UNIT()
SI_UNIT($,.RADIAN.)
);
#14129=(
NAMED_UNIT(*)
SI_UNIT($,.STERADIAN.)
SOLID_ANGLE_UNIT()
);
#14132=SHAPE_DEFINITION_REPRESENTATION(#14144,#14201);
#14144=PRODUCT_DEFINITION_SHAPE('',$,#14214);
#14201=SHAPE_REPRESENTATION('',(#6338),#14115);
#14211=PRODUCT_DEFINITION_CONTEXT('part definition',#14249,'design');
#14214=PRODUCT_DEFINITION('Back Lid','Back Lid',#14226,#14211);
#14226=PRODUCT_DEFINITION_FORMATION('',$,#14253);
#14249=APPLICATION_CONTEXT(
'Core Data for Automotive Mechanical Design Process');
#14250=PRODUCT_CONTEXT('part definition',#14249,'mechanical');
#14253=PRODUCT('Back Lid','Back Lid',$,(#14250));
#14263=PRESENTATION_STYLE_ASSIGNMENT((#14265));
#14265=SURFACE_STYLE_USAGE(.BOTH.,#14267);
#14267=SURFACE_SIDE_STYLE('',(#14269));
#14269=SURFACE_STYLE_FILL_AREA(#14271);
#14271=FILL_AREA_STYLE('Steel - Satin',(#14273));
#14273=FILL_AREA_STYLE_COLOUR('Steel - Satin',#14275);
#14275=COLOUR_RGB('Steel - Satin',0.627450980392157,0.627450980392157,0.627450980392157);
ENDSEC;
END-ISO-10303-21;
